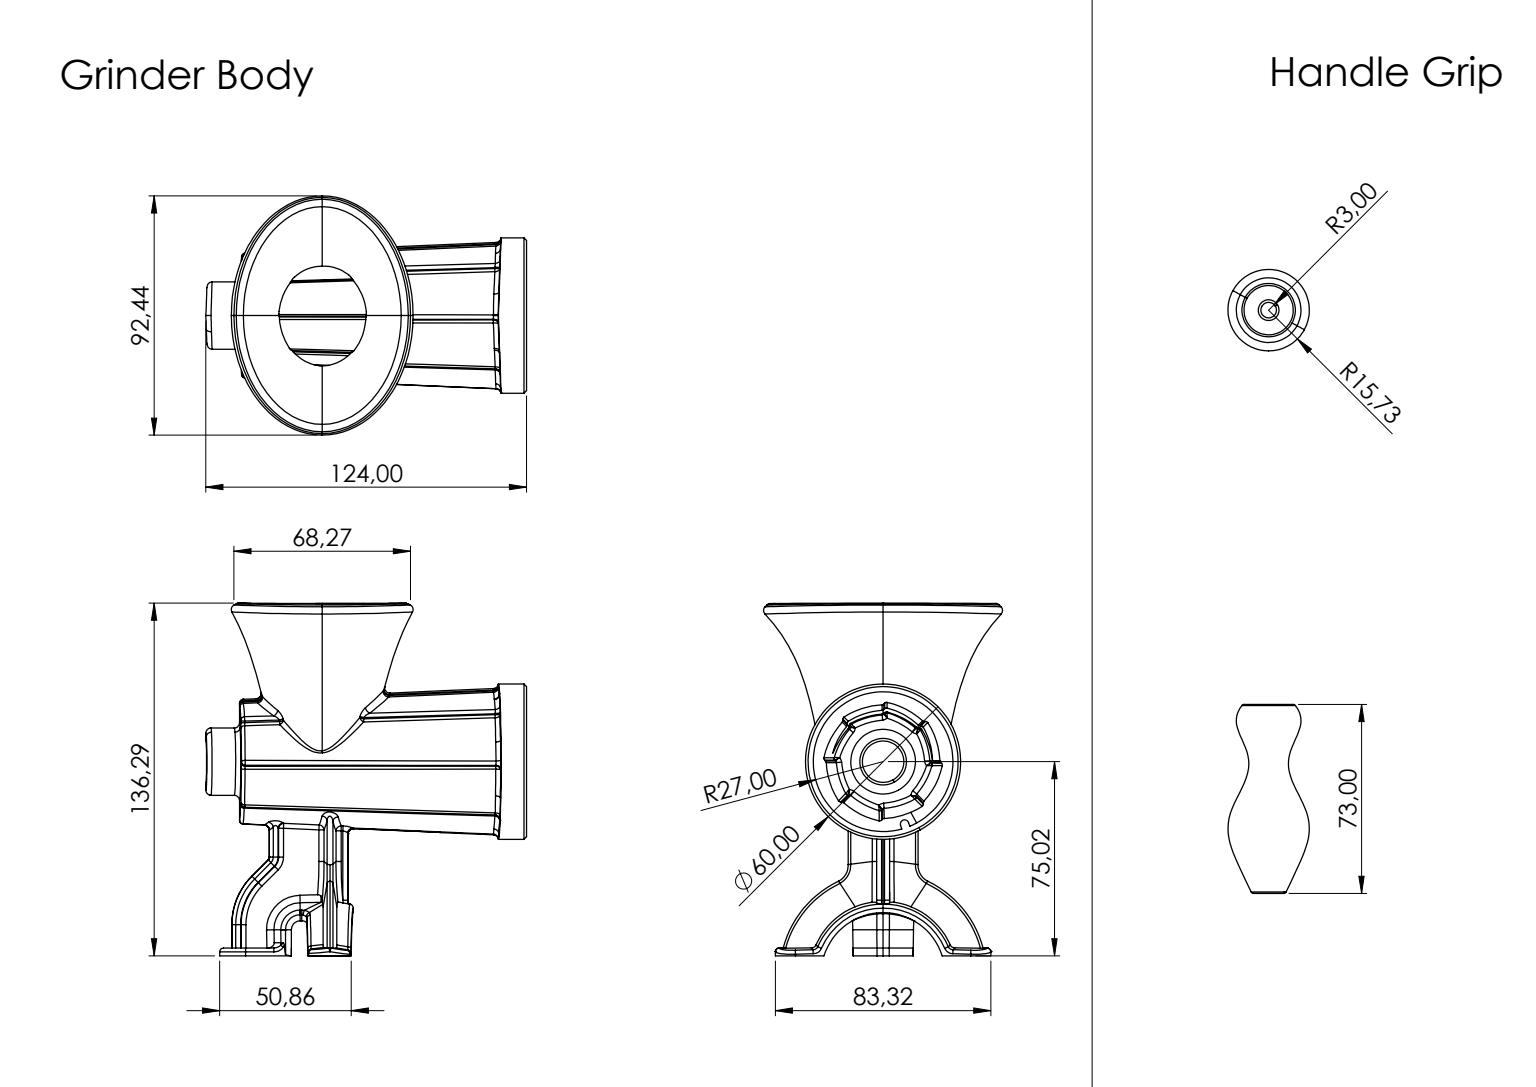
ISO-10303-21;
HEADER;
FILE_DESCRIPTION (('STEP AP214'),
    '1' );
FILE_NAME ('Handle Grip.step',
    '2026-10-06T09:49:54',
    ( '' ),
    ( '' ),
    'SwSTEP 2.0',
    'SolidWorks 2020',
    '' );
FILE_SCHEMA (( 'AUTOMOTIVE_DESIGN' ));
ENDSEC;

DATA;
#101=AXIS2_PLACEMENT_3D ( 'NONE', #52542, #86674, #33491 ) ;
#229=( LENGTH_UNIT ( ) NAMED_UNIT ( * ) SI_UNIT ( .MILLI., .METRE. ) );
#251=ORIENTED_EDGE ( 'NONE', *, *, #53107, .T. ) ;
#286=DIRECTION ( 'NONE',  ( 0.8775825618903774217, -3.365001152038843908E-31, 0.4794255386041944567 ) ) ;
#350=CARTESIAN_POINT ( 'NONE',  ( -113.4000000000000057, 1358.631207110790001, 311.1659210709989907 ) ) ;
#403=CIRCLE ( 'NONE', #27160, 5.868098490439995985 ) ;
#829=CARTESIAN_POINT ( 'NONE',  ( -113.4000000000000057, 1306.913060387289988, 304.2218459572590064 ) ) ;
#1026=AXIS2_PLACEMENT_3D ( 'NONE', #39081, #107399, #20087 ) ;
#1200=DIRECTION ( 'NONE',  ( -1.836970198721029688E-16, -1.000000000000000000, 0.000000000000000000 ) ) ;
#1407=VERTEX_POINT ( 'NONE', #25256 ) ;
#1429=CARTESIAN_POINT ( 'NONE',  ( -110.7672523143288856, 1378.813060387289852, 305.6601225730716465 ) ) ;
#1717=CARTESIAN_POINT ( 'NONE',  ( -113.4000000000000057, 1306.483669372790018, 297.4506287831990221 ) ) ;
#2006=CARTESIAN_POINT ( 'NONE',  ( -121.4211954113600029, 1309.112692017090239, 304.2218459572590064 ) ) ;
#2272=ORIENTED_EDGE ( 'NONE', *, *, #46910, .F. ) ;
#2632=VECTOR ( 'NONE', #26109, 1000.000000000000114 ) ;
#2857=VERTEX_POINT ( 'NONE', #4258 ) ;
#2858=AXIS2_PLACEMENT_3D ( 'NONE', #14026, #56057, #90747 ) ;
#2967=CARTESIAN_POINT ( 'NONE',  ( -113.4000000000000057, 1377.418846546390114, 293.0440248834589738 ) ) ;
#3089=EDGE_LOOP ( 'NONE', ( #34929, #47856, #37715, #44340, #103281 ) ) ;
#3113=CARTESIAN_POINT ( 'NONE',  ( -113.4000000000000057, 1306.483669372790018, 310.9930631313190474 ) ) ;
#3988=ORIENTED_EDGE ( 'NONE', *, *, #12337, .F. ) ;
#4058=CARTESIAN_POINT ( 'NONE',  ( -100.5161172129000136, 1371.894749952189613, 291.3379631701586732 ) ) ;
#4196=( LENGTH_UNIT ( ) NAMED_UNIT ( * ) SI_UNIT ( .MILLI., .METRE. ) );
#4258=CARTESIAN_POINT ( 'NONE',  ( -110.8380420702032580, 1377.913060387289988, 302.6609578876201567 ) ) ;
#4283=ORIENTED_EDGE ( 'NONE', *, *, #31051, .F. ) ;
#4332=CARTESIAN_POINT ( 'NONE',  ( -123.8569892972382007, 1368.558218059088176, 298.5091666679096534 ) ) ;
#4655=CARTESIAN_POINT ( 'NONE',  ( -113.4000000000000057, 1378.913060387289988, 304.2218459572590064 ) ) ;
#4738=CARTESIAN_POINT ( 'NONE',  ( -113.4000000000000057, 1377.913060387289988, 304.2218459572590064 ) ) ;
#5130=CARTESIAN_POINT ( 'NONE',  ( -113.4000000000000057, 1368.558218059089995, 292.3061701549589770 ) ) ;
#5132=DIRECTION ( 'NONE',  ( -1.836970198721029688E-16, -1.000000000000000000, 0.000000000000000000 ) ) ;
#5415=CARTESIAN_POINT ( 'NONE',  ( -124.5778210737999672, 1377.418846546389204, 315.3996670310588115 ) ) ;
#5523=ORIENTED_EDGE ( 'NONE', *, *, #44607, .T. ) ;
#5697=CARTESIAN_POINT ( 'NONE',  ( -113.4000000000000057, 1340.114449826970031, 286.9633900369479989 ) ) ;
#5970=CARTESIAN_POINT ( 'NONE',  ( -125.6580589596999431, 1375.179104070691892, 301.0918496320489339 ) ) ;
#6184=CARTESIAN_POINT ( 'NONE',  ( -113.4000000000000057, 1306.483669372790018, 304.2218459572590064 ) ) ;
#6228=CARTESIAN_POINT ( 'NONE',  ( -122.7580815721776446, 1314.643966242389979, 299.1095026942255686 ) ) ;
#6517=CARTESIAN_POINT ( 'NONE',  ( -130.6584559203111269, 1340.114449826969121, 299.8150386652596353 ) ) ;
#6581=DIRECTION ( 'NONE',  ( -0.4794255386041976763, 8.806904269216897590E-17, 0.8775825618903756453 ) ) ;
#6680=CARTESIAN_POINT ( 'NONE',  ( -102.9430107027000076, 1368.558218059089995, 309.9345252466190459 ) ) ;
#6772=CARTESIAN_POINT ( 'NONE',  ( -96.21470915085021147, 1331.448250124730293, 287.0365551081087574 ) ) ;
#6912=CARTESIAN_POINT ( 'NONE',  ( -123.3741145675100057, 1345.325269380309919, 298.7729623350389829 ) ) ;
#7070=CARTESIAN_POINT ( 'NONE',  ( -126.6653580272000283, 1320.102705746890024, 317.4872039844593132 ) ) ;
#7239=CARTESIAN_POINT ( 'NONE',  ( -107.4576978852700080, 1306.483669372790018, 307.4681403979390097 ) ) ;
#7336=CARTESIAN_POINT ( 'NONE',  ( -113.4000000000000057, 1348.229899472569969, 298.0159978832119805 ) ) ;
#7468=CARTESIAN_POINT ( 'NONE',  ( -125.0414468819000007, 1320.102705746890251, 297.8620945402790312 ) ) ;
#7518=DIRECTION ( 'NONE',  ( -1.836970198721029688E-16, -1.000000000000000000, 0.000000000000000000 ) ) ;
#7591=VERTEX_POINT ( 'NONE', #51464 ) ;
#7614=CARTESIAN_POINT ( 'NONE',  ( -119.4939992282754417, 1358.631207110788182, 300.8926790057471408 ) ) ;
#7900=ADVANCED_FACE ( 'NONE', ( #17152 ), #95557, .F. ) ;
#8015=CARTESIAN_POINT ( 'NONE',  ( -122.8636594665699988, 1366.350733876289951, 299.0518252276390285 ) ) ;
#8157=CARTESIAN_POINT ( 'NONE',  ( -125.0414468819037381, 1320.102705746890024, 297.8620945402922757 ) ) ;
#8706=DIRECTION ( 'NONE',  ( -1.836970198721029688E-16, -1.000000000000000000, -1.314768175368352060E-31 ) ) ;
#8707=CARTESIAN_POINT ( 'NONE',  ( -120.3440751137400042, 1358.631207110790001, 304.2218459572590064 ) ) ;
#8815=DIRECTION ( 'NONE',  ( -1.000000000000000000, 1.836970198721029688E-16, 0.000000000000000000 ) ) ;
#9133=APPLICATION_CONTEXT ( 'automotive_design' ) ;
#9933=PLANE ( 'NONE',  #92465 ) ;
#10275=VERTEX_POINT ( 'NONE', #42078 ) ;
#10464=EDGE_CURVE ( 'NONE', #44860, #89357, #58741, .T. ) ;
#10704=AXIS2_PLACEMENT_3D ( 'NONE', #108539, #65462, #107981 ) ;
#10869=VERTEX_POINT ( 'NONE', #110110 ) ;
#11071=DIRECTION ( 'NONE',  ( -4.648609652910299899E-17, -1.000000000000000000, 2.252106476759999926E-16 ) ) ;
#11095=AXIS2_PLACEMENT_3D ( 'NONE', #75738, #33162, #91434 ) ;
#11349=CARTESIAN_POINT ( 'NONE',  ( -101.5731991332999513, 1376.302340817389677, 292.3950450905593357 ) ) ;
#11561=CIRCLE ( 'NONE', #74167, 0.9999999999999930056 ) ;
#11756=PRODUCT_DEFINITION ( 'UNKNOWN', '', #20769, #12102 ) ;
#12085=DIRECTION ( 'NONE',  ( 0.4794255386041977873, -8.806904269216896357E-17, -0.8775825618903755343 ) ) ;
#12102=PRODUCT_DEFINITION_CONTEXT ( 'detailed design', #9133, 'design' ) ;
#12158=( GEOMETRIC_REPRESENTATION_CONTEXT ( 3 ) GLOBAL_UNCERTAINTY_ASSIGNED_CONTEXT ( ( #92795 ) ) GLOBAL_UNIT_ASSIGNED_CONTEXT ( ( #4196, #29376, #13113 ) ) REPRESENTATION_CONTEXT ( 'NONE', 'WORKASPACE' ) );
#12337=EDGE_CURVE ( 'NONE', #26502, #73768, #403, .T. ) ;
#12429=CARTESIAN_POINT ( 'NONE',  ( -101.1419410403000541, 1375.179104070690755, 291.9637869975591684 ) ) ;
#12459=ADVANCED_FACE ( 'NONE', ( #31711 ), #24972, .T. ) ;
#12466=ORIENTED_EDGE ( 'NONE', *, *, #70639, .F. ) ;
#12558=EDGE_CURVE ( 'NONE', #2857, #32152, #104036, .T. ) ;
#12715=CARTESIAN_POINT ( 'NONE',  ( -125.2268008667000743, 1376.302340817389677, 301.2019679020577883 ) ) ;
#12885=AXIS2_PLACEMENT_3D ( 'NONE', #6184, #77810, #102438 ) ;
#12969=CARTESIAN_POINT ( 'NONE',  ( -102.2221789262000016, 1377.418846546389659, 307.0760123268498205 ) ) ;
#12970=CARTESIAN_POINT ( 'NONE',  ( -113.4000000000000057, 1378.913060387289988, 304.2218459572590064 ) ) ;
#13113=( NAMED_UNIT ( * ) SI_UNIT ( $, .STERADIAN. ) SOLID_ANGLE_UNIT ( ) );
#13511=CARTESIAN_POINT ( 'NONE',  ( -102.6162175075999983, 1366.350733876289951, 304.2218459572590064 ) ) ;
#13792=CARTESIAN_POINT ( 'NONE',  ( -123.2094608542982570, 1377.418846546388068, 298.8629130685321229 ) ) ;
#14026=CARTESIAN_POINT ( 'NONE',  ( -113.4000000000000057, 1377.913060387289988, 304.2218459572590064 ) ) ;
#14069=CARTESIAN_POINT ( 'NONE',  ( -113.4000000000000057, 1358.631207110790001, 297.2777708435189652 ) ) ;
#14451=CARTESIAN_POINT ( 'NONE',  ( -115.9619579297967391, 1377.913060387289988, 305.7827340268977991 ) ) ;
#14606=MECHANICAL_DESIGN_GEOMETRIC_PRESENTATION_REPRESENTATION('',(#39642),#34280);
#14628=CARTESIAN_POINT ( 'NONE',  ( -98.25428012471454053, 1340.114449826970258, 312.4959906388990589 ) ) ;
#14643=ORIENTED_EDGE ( 'NONE', *, *, #65595, .F. ) ;
#14862=DIRECTION ( 'NONE',  ( 0.8775825618903687619, 0.000000000000000000, 0.4794255386042102218 ) ) ;
#14900=CARTESIAN_POINT ( 'NONE',  ( -113.4000000000000057, 1320.102705746890251, 317.4872039844590290 ) ) ;
#14956=DIRECTION ( 'NONE',  ( 0.8775825618903754233, 0.000000000000000000, 0.4794255386041978984 ) ) ;
#15074=ORIENTED_EDGE ( 'NONE', *, *, #108277, .F. ) ;
#15161=CARTESIAN_POINT ( 'NONE',  ( -101.4843241977000758, 1368.558218059089995, 292.3061701549589770 ) ) ;
#15290=ORIENTED_EDGE ( 'NONE', *, *, #102111, .T. ) ;
#15299=CARTESIAN_POINT ( 'NONE',  ( -127.5184075663999863, 1336.950374720429863, 296.5089247511289727 ) ) ;
#15448=CARTESIAN_POINT ( 'NONE',  ( -124.1837824923999989, 1366.350733876289951, 304.2218459572590064 ) ) ;
#15582=ORIENTED_EDGE ( 'NONE', *, *, #104815, .T. ) ;
#15601=CARTESIAN_POINT ( 'NONE',  ( -102.0933291366000049, 1371.894749952190068, 310.3987084017590519 ) ) ;
#15700=CARTESIAN_POINT ( 'NONE',  ( -104.0419184806740134, 1314.643966242388842, 309.3341893170371577 ) ) ;
#15995=CARTESIAN_POINT ( 'NONE',  ( -119.6058480740469463, 1348.229899472570878, 302.6372327872264236 ) ) ;
#16163=CARTESIAN_POINT ( 'NONE',  ( -100.0318980807000031, 1325.797319984390015, 311.5248733202390099 ) ) ;
#16227=CARTESIAN_POINT ( 'NONE',  ( -105.0428569062679145, 1377.913060387289988, 308.7873740373456144 ) ) ;
#16321=CARTESIAN_POINT ( 'NONE',  ( -113.4000000000000057, 1308.913060387289988, 304.2218459572590064 ) ) ;
#16535=CARTESIAN_POINT ( 'NONE',  ( -120.3440751137400895, 1358.631207110789774, 311.1659210709988770 ) ) ;
#16780=CARTESIAN_POINT ( 'NONE',  ( -113.4000000000000057, 1375.913060387289988, 304.2218459572590064 ) ) ;
#17081=CARTESIAN_POINT ( 'NONE',  ( -128.5457199608194401, 1340.114449826969576, 295.9477014321888646 ) ) ;
#17152=FACE_OUTER_BOUND ( 'NONE', #3089, .T. ) ;
#17255=CARTESIAN_POINT ( 'NONE',  ( -99.28159243359999664, 1336.950374720429863, 311.9347671633890400 ) ) ;
#17443=AXIS2_PLACEMENT_3D ( 'NONE', #30561, #73124, #54692 ) ;
#17475=DIRECTION ( 'NONE',  ( 9.404037925578970303E-16, -1.000000000000000000, 2.220446049250000002E-16 ) ) ;
#17505=ORIENTED_EDGE ( 'NONE', *, *, #35220, .F. ) ;
#17543=VERTEX_POINT ( 'NONE', #37700 ) ;
#17810=CARTESIAN_POINT ( 'NONE',  ( -105.2220349633299890, 1311.832804576489934, 308.6894886186490226 ) ) ;
#17819=VERTEX_POINT ( 'NONE', #74067 ) ;
#18298=DIRECTION ( 'NONE',  ( -1.836970198721029688E-16, -1.000000000000000000, 0.000000000000000000 ) ) ;
#18816=LINE ( 'NONE', #45167, #2632 ) ;
#18866=DIRECTION ( 'NONE',  ( -1.836970198721029688E-16, -1.000000000000000000, 0.000000000000000000 ) ) ;
#19178=SURFACE_STYLE_FILL_AREA ( #70212 ) ;
#19307=CARTESIAN_POINT ( 'NONE',  ( -120.1712171740600041, 1306.483669372790018, 304.2218459572590064 ) ) ;
#19407=EDGE_CURVE ( 'NONE', #20038, #77300, #65776, .T. ) ;
#19502=CARTESIAN_POINT ( 'NONE',  ( -113.4000000000000057, 1375.913060387289988, 304.2218459572590064 ) ) ;
#19593=DIRECTION ( 'NONE',  ( 0.8775825618903774217, -3.365001152038843908E-31, 0.4794255386041944567 ) ) ;
#19696=VERTEX_POINT ( 'NONE', #44493 ) ;
#20038=VERTEX_POINT ( 'NONE', #73706 ) ;
#20087=DIRECTION ( 'NONE',  ( -1.000000000000000000, 1.836970198721029688E-16, 0.000000000000000000 ) ) ;
#20173=DIRECTION ( 'NONE',  ( -1.000000000000000000, 0.000000000000000000, 0.000000000000000000 ) ) ;
#20271=CARTESIAN_POINT ( 'NONE',  ( -113.4000000000000057, 1378.528619065190014, 293.9108410952590020 ) ) ;
#20435=EDGE_CURVE ( 'NONE', #77300, #38227, #60419, .T. ) ;
#20538=ORIENTED_EDGE ( 'NONE', *, *, #12337, .T. ) ;
#20769=PRODUCT_DEFINITION_FORMATION_WITH_SPECIFIED_SOURCE ( 'ANY', '', #39314, .NOT_KNOWN. ) ;
#20819=CARTESIAN_POINT ( 'NONE',  ( -102.2221789262000726, 1377.418846546389204, 293.0440248834591443 ) ) ;
#20974=FACE_OUTER_BOUND ( 'NONE', #64827, .T. ) ;
#21092=CARTESIAN_POINT ( 'NONE',  ( -125.2268008667000174, 1376.302340817389904, 304.2218459572590064 ) ) ;
#21151=CIRCLE ( 'NONE', #57012, 0.9999999999999930056 ) ;
#21355=CARTESIAN_POINT ( 'NONE',  ( -102.6425412750940325, 1375.179104070689846, 310.0986725874599870 ) ) ;
#21632=AXIS2_PLACEMENT_3D ( 'NONE', #110085, #42890, #42328 ) ;
#21717=FACE_OUTER_BOUND ( 'NONE', #33987, .T. ) ;
#21901=CARTESIAN_POINT ( 'NONE',  ( -102.7365228771000005, 1314.643966242390206, 304.2218459572590064 ) ) ;
#22452=CARTESIAN_POINT ( 'NONE',  ( -106.4559248862599361, 1358.631207110789774, 297.2777708435190220 ) ) ;
#22482=ORIENTED_EDGE ( 'NONE', *, *, #31051, .T. ) ;
#22521=DIRECTION ( 'NONE',  ( -1.836970198721029688E-16, -1.000000000000000000, -1.314768175368352060E-31 ) ) ;
#22735=CARTESIAN_POINT ( 'NONE',  ( -103.0210057964301740, 1376.302340817391269, 309.8919163327337856 ) ) ;
#23017=CARTESIAN_POINT ( 'NONE',  ( -107.3060008061400197, 1358.631207110790911, 307.5510129717682162 ) ) ;
#23093=LINE ( 'NONE', #90859, #65252 ) ;
#23162=VECTOR ( 'NONE', #70390, 1000.000000000000227 ) ;
#23304=CARTESIAN_POINT ( 'NONE',  ( -125.3156758022999213, 1368.558218059088631, 301.1792744052535227 ) ) ;
#23576=CARTESIAN_POINT ( 'NONE',  ( -106.3607388212290061, 1309.112692017090239, 308.0674119603681902 ) ) ;
#23848=CARTESIAN_POINT ( 'NONE',  ( -107.8722023357835695, 1311.832804576487888, 313.5405874544188123 ) ) ;
#23924=LINE ( 'NONE', #48056, #38012 ) ;
#24111=CARTESIAN_POINT ( 'NONE',  ( -120.4682768577266927, 1368.558218059088176, 292.3061701549587497 ) ) ;
#24405=CARTESIAN_POINT ( 'NONE',  ( -124.1837824924000557, 1366.350733876290406, 301.4682942176205529 ) ) ;
#24627=ADVANCED_FACE ( 'NONE', ( #64326, #21717 ), #71653, .F. ) ;
#24835=AXIS2_PLACEMENT_3D ( 'NONE', #19502, #53704, #87845 ) ;
#24899=DIRECTION ( 'NONE',  ( -1.000000000000000000, 0.000000000000000000, 0.000000000000000000 ) ) ;
#24911=ORIENTED_EDGE ( 'NONE', *, *, #44245, .T. ) ;
#24939=CARTESIAN_POINT ( 'NONE',  ( -125.3156758022999924, 1368.558218059089995, 304.2218459572590064 ) ) ;
#24972=( BOUNDED_SURFACE ( )  B_SPLINE_SURFACE ( 5, 2, ( 
 ( #91066, #64807, #98915, #107324, #82679, #56385, #106226 ),
 ( #13792, #47976, #82116, #5415, #39574, #46352, #40115 ),
 ( #73747, #12715, #21092, #107871, #38462, #99457, #22735 ),
 ( #65897, #5970, #100014, #54747, #88877, #37930, #72112 ),
 ( #29510, #63703, #46899, #55295, #97813, #89425, #81023 ),
 ( #4332, #23304, #24939, #34477, #108987, #59151, #109536 ),
 ( #32810, #24405, #15448, #93804, #58039, #66995, #76477 ),
 ( #7614, #93272, #8707, #16535, #350, #83227, #85408 ),
 ( #50726, #15995, #49639, #84323, #101105, #41227, #75397 ),
 ( #17081, #6517, #25502, #67550, #50197, #40670, #42885 ),
 ( #83776, #84857, #92177, #57499, #41770, #75927, #58589 ),
 ( #8157, #32272, #42324, #7070, #14900, #66454, #74843 ),
 ( #92719, #91624, #77042, #59692, #110080, #33356, #101652 ),
 ( #51276, #110630, #100567, #33913, #68107, #23848, #102222 ),
 ( #68652, #49092, #2006, #103884, #37242, #96036, #36141 ),
 ( #104438, #35572, #19307, #35021, #3113, #79254, #26048 ) ),
 .UNSPECIFIED., .F., .F., .F. ) 
 B_SPLINE_SURFACE_WITH_KNOTS ( ( 6, 3, 3, 1, 3, 6 ),
 ( 3, 2, 2, 3 ),
 ( 0.4214913904879999951, 6.500000000000000000, 18.08975840989999995, 46.86861349480000172, 60.45619974110000072, 75.86994138869999915 ),
 ( 2.628620570832299830, 3.141592653589790007, 4.712388980384689674, 5.770213224422659160 ),
 .UNSPECIFIED. ) 
 GEOMETRIC_REPRESENTATION_ITEM ( )  RATIONAL_B_SPLINE_SURFACE ( (
 ( 0.8711730262222689980, 0.9043503973638329363, 1.000000000000000000, 0.7071067811865480168, 1.000000000000000000, 0.8027563838226099424, 0.8711730262223420507),
 ( 0.8711730262222689980, 0.9043503973638329363, 1.000000000000000000, 0.7071067811865480168, 1.000000000000000000, 0.8027563838226099424, 0.8711730262223420507),
 ( 0.8711730262222689980, 0.9043503973638329363, 1.000000000000000000, 0.7071067811865480168, 1.000000000000000000, 0.8027563838226099424, 0.8711730262223420507),
 ( 0.8711730262222689980, 0.9043503973638329363, 1.000000000000000000, 0.7071067811865480168, 1.000000000000000000, 0.8027563838226099424, 0.8711730262223420507),
 ( 0.8711730262222689980, 0.9043503973638329363, 1.000000000000000000, 0.7071067811865480168, 1.000000000000000000, 0.8027563838226099424, 0.8711730262223420507),
 ( 0.8711730262222689980, 0.9043503973638329363, 1.000000000000000000, 0.7071067811865480168, 1.000000000000000000, 0.8027563838226099424, 0.8711730262223420507),
 ( 0.8711730262222689980, 0.9043503973638329363, 1.000000000000000000, 0.7071067811865480168, 1.000000000000000000, 0.8027563838226099424, 0.8711730262223420507),
 ( 0.8711730262222689980, 0.9043503973638329363, 1.000000000000000000, 0.7071067811865480168, 1.000000000000000000, 0.8027563838226099424, 0.8711730262223420507),
 ( 0.8711730262222689980, 0.9043503973638329363, 1.000000000000000000, 0.7071067811865480168, 1.000000000000000000, 0.8027563838226099424, 0.8711730262223420507),
 ( 0.8711730262222689980, 0.9043503973638329363, 1.000000000000000000, 0.7071067811865480168, 1.000000000000000000, 0.8027563838226099424, 0.8711730262223420507),
 ( 0.8711730262222689980, 0.9043503973638329363, 1.000000000000000000, 0.7071067811865480168, 1.000000000000000000, 0.8027563838226099424, 0.8711730262223420507),
 ( 0.8711730262222689980, 0.9043503973638329363, 1.000000000000000000, 0.7071067811865480168, 1.000000000000000000, 0.8027563838226099424, 0.8711730262223420507),
 ( 0.8711730262222689980, 0.9043503973638329363, 1.000000000000000000, 0.7071067811865480168, 1.000000000000000000, 0.8027563838226099424, 0.8711730262223420507),
 ( 0.8711730262222689980, 0.9043503973638329363, 1.000000000000000000, 0.7071067811865480168, 1.000000000000000000, 0.8027563838226099424, 0.8711730262223420507),
 ( 0.8711730262222689980, 0.9043503973638329363, 1.000000000000000000, 0.7071067811865480168, 1.000000000000000000, 0.8027563838226099424, 0.8711730262223420507),
 ( 0.8711730262222689980, 0.9043503973638329363, 1.000000000000000000, 0.7071067811865480168, 1.000000000000000000, 0.8027563838226099424, 0.8711730262223420507) ) ) 
 REPRESENTATION_ITEM ( '' )  SURFACE ( )  );
#25213=CARTESIAN_POINT ( 'NONE',  ( -113.4000000000000057, 1309.112692017090239, 296.2006505458990091 ) ) ;
#25256=CARTESIAN_POINT ( 'NONE',  ( -119.3423021147300034, 1306.483669372790018, 300.9755515165790030 ) ) ;
#25349=CARTESIAN_POINT ( 'NONE',  ( -127.3242238164999947, 1328.501055712589960, 296.6150078171390305 ) ) ;
#25444=EDGE_CURVE ( 'NONE', #10869, #2857, #51125, .T. ) ;
#25502=CARTESIAN_POINT ( 'NONE',  ( -130.6584559203110132, 1340.114449826970031, 304.2218459572590064 ) ) ;
#25523=ORIENTED_EDGE ( 'NONE', *, *, #12558, .T. ) ;
#26048=CARTESIAN_POINT ( 'NONE',  ( -107.4576978852700648, 1306.483669372788427, 307.4681403979344623 ) ) ;
#26109=DIRECTION ( 'NONE',  ( -0.6038592750913972518, 0.7071067811868648745, 0.3679048462383220919 ) ) ;
#26295=DIRECTION ( 'NONE',  ( 0.4794255386042002298, -8.806904269216945661E-17, -0.8775825618903744241 ) ) ;
#26502=VERTEX_POINT ( 'NONE', #109208 ) ;
#26555=DIRECTION ( 'NONE',  ( -4.222254822704919979E-17, -1.000000000000000000, 7.728785610902649958E-17 ) ) ;
#27122=CONICAL_SURFACE ( 'NONE', #39661, 0.9999999999999956701, 0.7853981633970000820 ) ;
#27160=AXIS2_PLACEMENT_3D ( 'NONE', #68239, #59824, #77175 ) ;
#27610=SHAPE_REPRESENTATION_RELATIONSHIP ( 'NONE' , 'NONE' ,  #45156, #67999 ) ;
#27847=CARTESIAN_POINT ( 'NONE',  ( -106.8999999999999915, 1305.913060387289988, 304.2218459572590064 ) ) ;
#28228=STYLED_ITEM ( 'NONE', ( #87654 ), #46097 ) ;
#28303=EDGE_CURVE ( 'NONE', #17819, #38227, #106482, .T. ) ;
#28529=AXIS2_PLACEMENT_3D ( 'NONE', #4738, #98798, #105568 ) ;
#28846=FILL_AREA_STYLE_COLOUR ( '', #76500 ) ;
#28896=CIRCLE ( 'NONE', #44985, 0.9999999999999930056 ) ;
#28917=UNCERTAINTY_MEASURE_WITH_UNIT (LENGTH_MEASURE( 1.000000000000000082E-05 ), #80223, 'distance_accuracy_value', 'NONE');
#28977=DIRECTION ( 'NONE',  ( -1.000000000000000000, 0.000000000000000000, 0.000000000000000000 ) ) ;
#29376=( NAMED_UNIT ( * ) PLANE_ANGLE_UNIT ( ) SI_UNIT ( $, .RADIAN. ) );
#29510=CARTESIAN_POINT ( 'NONE',  ( -124.7066708633992391, 1371.894749952189386, 298.0449835127411689 ) ) ;
#29511=EDGE_CURVE ( 'NONE', #38227, #17543, #42104, .T. ) ;
#29747=ORIENTED_EDGE ( 'NONE', *, *, #82319, .T. ) ;
#29782=CARTESIAN_POINT ( 'NONE',  ( -103.0889951380000156, 1378.528619065190696, 293.9108410952588883 ) ) ;
#30156=ORIENTED_EDGE ( 'NONE', *, *, #108277, .T. ) ;
#30561=CARTESIAN_POINT ( 'NONE',  ( -113.4000000000000057, 1378.913060387289988, 304.2218459572590064 ) ) ;
#30575=CYLINDRICAL_SURFACE ( 'NONE', #90237, 3.000000000000017764 ) ;
#30696=ORIENTED_EDGE ( 'NONE', *, *, #65845, .T. ) ;
#30877=CARTESIAN_POINT ( 'NONE',  ( -122.8636594665523489, 1366.350733876290178, 299.0518252276563658 ) ) ;
#30977=EDGE_CURVE ( 'NONE', #81044, #19696, #18816, .T. ) ;
#31051=EDGE_CURVE ( 'NONE', #17819, #73768, #11561, .T. ) ;
#31052=ORIENTED_EDGE ( 'NONE', *, *, #65845, .F. ) ;
#31430=CARTESIAN_POINT ( 'NONE',  ( -107.1941519259529230, 1348.229899472571105, 305.8064591614598839 ) ) ;
#31711=FACE_OUTER_BOUND ( 'NONE', #80783, .T. ) ;
#31985=CARTESIAN_POINT ( 'NONE',  ( -113.4000000000000057, 1311.832804576489934, 294.9031044600990299 ) ) ;
#32123=CARTESIAN_POINT ( 'NONE',  ( -119.0092909768300018, 1350.849221539110204, 301.1574763303589748 ) ) ;
#32152=VERTEX_POINT ( 'NONE', #63754 ) ;
#32272=CARTESIAN_POINT ( 'NONE',  ( -126.6653580271998862, 1320.102705746891161, 300.8346439529095164 ) ) ;
#32545=CARTESIAN_POINT ( 'NONE',  ( -98.31848851494262931, 1331.448250124730066, 312.4609134345859047 ) ) ;
#32810=CARTESIAN_POINT ( 'NONE',  ( -122.8636594665494499, 1366.350733876287677, 299.0518252276506814 ) ) ;
#32974=CARTESIAN_POINT ( 'NONE',  ( -107.3060007717200079, 1358.631207110790001, 307.5510129087689961 ) ) ;
#33078=CARTESIAN_POINT ( 'NONE',  ( -103.9363405868959518, 1366.350733876290633, 309.3918667846981521 ) ) ;
#33145=EDGE_CURVE ( 'NONE', #2857, #7591, #23924, .T. ) ;
#33162=DIRECTION ( 'NONE',  ( -1.836970198721029688E-16, -1.000000000000000000, 0.000000000000000000 ) ) ;
#33215=CARTESIAN_POINT ( 'NONE',  ( -122.4487580624700058, 1378.528619065190014, 299.2784868977390147 ) ) ;
#33356=CARTESIAN_POINT ( 'NONE',  ( -107.0745166769187335, 1314.643966242389979, 314.8853230801587415 ) ) ;
#33491=DIRECTION ( 'NONE',  ( -1.000000000000000000, 0.000000000000000000, 0.000000000000000000 ) ) ;
#33513=CARTESIAN_POINT ( 'NONE',  ( -104.3512419375300055, 1378.528619065190014, 309.1652050167789980 ) ) ;
#33657=AXIS2_PLACEMENT_3D ( 'NONE', #94224, #69069, #42188 ) ;
#33913=CARTESIAN_POINT ( 'NONE',  ( -122.7187414971600390, 1311.832804576490389, 313.5405874544188691 ) ) ;
#33987=EDGE_LOOP ( 'NONE', ( #15074, #51270 ) ) ;
#34206=CLOSED_SHELL ( 'NONE', ( #74966, #61184, #92370, #7900, #41766, #53548, #66841, #98059, #103639, #24627, #76834, #93325, #12459, #91525 ) ) ;
#34280=( GEOMETRIC_REPRESENTATION_CONTEXT ( 3 ) GLOBAL_UNCERTAINTY_ASSIGNED_CONTEXT ( ( #28917 ) ) GLOBAL_UNIT_ASSIGNED_CONTEXT ( ( #80223, #71870, #80776 ) ) REPRESENTATION_CONTEXT ( 'NONE', 'WORKASPACE' ) );
#34339=ORIENTED_EDGE ( 'NONE', *, *, #33145, .T. ) ;
#34477=CARTESIAN_POINT ( 'NONE',  ( -125.3156758023000918, 1368.558218059089995, 316.1375217595589220 ) ) ;
#34541=CARTESIAN_POINT ( 'NONE',  ( -113.4000000000000057, 1378.813060387289852, 304.2218459572590064 ) ) ;
#34564=CARTESIAN_POINT ( 'NONE',  ( -113.4000000000000057, 1305.913060387289988, 304.2218459572590064 ) ) ;
#34643=CARTESIAN_POINT ( 'NONE',  ( -103.4258854324899914, 1345.325269380309919, 309.6707295794789729 ) ) ;
#34739=CARTESIAN_POINT ( 'NONE',  ( -107.4576979188310162, 1306.483669372790018, 307.4681404593670777 ) ) ;
#34929=ORIENTED_EDGE ( 'NONE', *, *, #25444, .F. ) ;
#35021=CARTESIAN_POINT ( 'NONE',  ( -120.1712171740600326, 1306.483669372790246, 310.9930631313191043 ) ) ;
#35220=EDGE_CURVE ( 'NONE', #17819, #1407, #48666, .T. ) ;
#35323=ORIENTED_EDGE ( 'NONE', *, *, #105278, .F. ) ;
#35572=CARTESIAN_POINT ( 'NONE',  ( -120.1712171740599473, 1306.483669372790928, 302.4928703550302203 ) ) ;
#35647=UNCERTAINTY_MEASURE_WITH_UNIT (LENGTH_MEASURE( 1.000000000000000082E-05 ), #229, 'distance_accuracy_value', 'NONE');
#35686=FACE_BOUND ( 'NONE', #108423, .T. ) ;
#35856=CARTESIAN_POINT ( 'NONE',  ( -118.1581044363824731, 1309.112692017089103, 296.2006505458993502 ) ) ;
#35876=DIRECTION ( 'NONE',  ( -0.4794255386042000078, 8.806904269216944428E-17, 0.8775825618903743131 ) ) ;
#36141=CARTESIAN_POINT ( 'NONE',  ( -106.3607387814725911, 1309.112692017088648, 308.0674118875946874 ) ) ;
#36160=ORIENTED_EDGE ( 'NONE', *, *, #35220, .T. ) ;
#36206=LINE ( 'NONE', #43510, #23162 ) ;
#36560=( NAMED_UNIT ( * ) PLANE_ANGLE_UNIT ( ) SI_UNIT ( $, .RADIAN. ) );
#37111=( NAMED_UNIT ( * ) SI_UNIT ( $, .STERADIAN. ) SOLID_ANGLE_UNIT ( ) );
#37207=FACE_OUTER_BOUND ( 'NONE', #75821, .T. ) ;
#37242=CARTESIAN_POINT ( 'NONE',  ( -113.4000000000000057, 1309.112692017090239, 312.2430413686190036 ) ) ;
#37700=CARTESIAN_POINT ( 'NONE',  ( -122.4487580624700058, 1378.528619065190014, 299.2784868977390147 ) ) ;
#37715=ORIENTED_EDGE ( 'NONE', *, *, #93623, .T. ) ;
#37924=EDGE_LOOP ( 'NONE', ( #108288, #20538 ) ) ;
#37930=CARTESIAN_POINT ( 'NONE',  ( -106.1286243849658177, 1375.179104070688027, 316.4799049169590717 ) ) ;
#38012=VECTOR ( 'NONE', #73821, 999.9999999999998863 ) ;
#38195=ORIENTED_EDGE ( 'NONE', *, *, #29511, .T. ) ;
#38227=VERTEX_POINT ( 'NONE', #76475 ) ;
#38462=CARTESIAN_POINT ( 'NONE',  ( -113.4000000000000057, 1376.302340817389904, 316.0486468239590181 ) ) ;
#38658=ORIENTED_EDGE ( 'NONE', *, *, #20435, .F. ) ;
#39071=AXIS2_PLACEMENT_3D ( 'NONE', #4655, #75180, #91421 ) ;
#39081=CARTESIAN_POINT ( 'NONE',  ( -103.4000000000000057, 1378.913060387289988, 304.2218459572590064 ) ) ;
#39286=CARTESIAN_POINT ( 'NONE',  ( -118.8461440515266929, 1348.229899472570651, 301.2466039018671609 ) ) ;
#39314=PRODUCT ( 'Handle Grip', 'Handle Grip', '', ( #73484 ) ) ;
#39478=EDGE_LOOP ( 'NONE', ( #95080, #25523, #60146, #42896, #31052 ) ) ;
#39568=ORIENTED_EDGE ( 'NONE', *, *, #93623, .F. ) ;
#39574=CARTESIAN_POINT ( 'NONE',  ( -113.4000000000000057, 1377.418846546390114, 315.3996670310589820 ) ) ;
#39576=EDGE_CURVE ( 'NONE', #10869, #41956, #23093, .T. ) ;
#39642=STYLED_ITEM ( 'NONE', ( #55041 ), #67999 ) ;
#39661=AXIS2_PLACEMENT_3D ( 'NONE', #16780, #69459, #49882 ) ;
#39842=CARTESIAN_POINT ( 'NONE',  ( -102.7365228771000574, 1314.643966242390661, 306.9446787514269204 ) ) ;
#40115=CARTESIAN_POINT ( 'NONE',  ( -103.5905391456986706, 1377.418846546389432, 309.5807788459800349 ) ) ;
#40274=CARTESIAN_POINT ( 'NONE',  ( -105.0428569062679145, 1378.913060387289988, 308.7873740373456144 ) ) ;
#40383=CARTESIAN_POINT ( 'NONE',  ( -125.0414468819076461, 1320.102705746891161, 297.8620945402992106 ) ) ;
#40670=CARTESIAN_POINT ( 'NONE',  ( -103.1624317239240867, 1340.114449826968666, 321.4803018775698433 ) ) ;
#40732=AXIS2_PLACEMENT_3D ( 'NONE', #16227, #26295, #42014 ) ;
#40834=CARTESIAN_POINT ( 'NONE',  ( -107.7907090231699954, 1350.849221539110204, 307.2862155841589811 ) ) ;
#40841=ORIENTED_EDGE ( 'NONE', *, *, #105278, .T. ) ;
#40936=CARTESIAN_POINT ( 'NONE',  ( -100.1346419727999972, 1320.102705746890251, 304.2218459572590064 ) ) ;
#41003=AXIS2_PLACEMENT_3D ( 'NONE', #87490, #17475, #103148 ) ;
#41069=CARTESIAN_POINT ( 'NONE',  ( -119.4939992282800034, 1358.631207110790001, 300.8926790057490166 ) ) ;
#41101=B_SPLINE_CURVE_WITH_KNOTS ( 'NONE', 5,
 ( #100960, #65738, #92564, #76894, #7468, #102066, #25349, #15299, #6912, #32123, #41069, #8015, #84168, #75784, #57355, #67404, #91480, #33215 ),
 .UNSPECIFIED., .F., .F.,
 ( 6, 3, 3, 3, 3, 6 ),
 ( -75.86994138869999915, -60.45619974110000072, -46.86861349480000172, -18.08975840989999284, -6.500000000000000000, -0.4214913904880006612 ),
 .UNSPECIFIED. ) ;
#41227=CARTESIAN_POINT ( 'NONE',  ( -109.7187440601658466, 1348.229899472568604, 310.4276940313056343 ) ) ;
#41399=CARTESIAN_POINT ( 'NONE',  ( -99.47577618349998829, 1328.501055712589960, 311.8286840973790390 ) ) ;
#41500=CARTESIAN_POINT ( 'NONE',  ( -96.14154407968899818, 1340.114449826970940, 286.9633900369476578 ) ) ;
#41766=ADVANCED_FACE ( 'NONE', ( #62881 ), #89285, .F. ) ;
#41770=CARTESIAN_POINT ( 'NONE',  ( -113.4000000000000057, 1331.448250124730066, 321.4071368064089711 ) ) ;
#41956=VERTEX_POINT ( 'NONE', #52513 ) ;
#42014=DIRECTION ( 'NONE',  ( -0.8775825618903754233, 0.000000000000000000, -0.4794255386041978984 ) ) ;
#42078=CARTESIAN_POINT ( 'NONE',  ( -116.9103302475592301, 1305.913060387289988, 302.3041438028434413 ) ) ;
#42104=CIRCLE ( 'NONE', #54674, 10.31100486199999722 ) ;
#42188=DIRECTION ( 'NONE',  ( -1.000000000000000000, 0.000000000000000000, 0.000000000000000000 ) ) ;
#42318=ORIENTED_EDGE ( 'NONE', *, *, #46910, .T. ) ;
#42324=CARTESIAN_POINT ( 'NONE',  ( -126.6653580271999999, 1320.102705746890251, 304.2218459572590064 ) ) ;
#42328=DIRECTION ( 'NONE',  ( 1.000000000000000000, 0.000000000000000000, 0.000000000000000000 ) ) ;
#42631=CIRCLE ( 'NONE', #33657, 10.31100486199999722 ) ;
#42838=TOROIDAL_SURFACE ( 'NONE', #28529, 9.522913805089999073, 1.000000000000000000 ) ;
#42885=CARTESIAN_POINT ( 'NONE',  ( -98.25428003917552644, 1340.114449826969576, 312.4959904823201100 ) ) ;
#42890=DIRECTION ( 'NONE',  ( 0.000000000000000000, 0.000000000000000000, 1.000000000000000000 ) ) ;
#42896=ORIENTED_EDGE ( 'NONE', *, *, #30977, .T. ) ;
#42979=DIRECTION ( 'NONE',  ( -1.000000000000000000, 0.000000000000000000, 0.000000000000000000 ) ) ;
#43510=CARTESIAN_POINT ( 'NONE',  ( -114.2775825618903696, 1308.913060387289988, 303.7424204186547740 ) ) ;
#44245=EDGE_CURVE ( 'NONE', #81044, #10869, #58749, .T. ) ;
#44340=ORIENTED_EDGE ( 'NONE', *, *, #44607, .F. ) ;
#44493=CARTESIAN_POINT ( 'NONE',  ( -116.8159439063953045, 1378.913060387289988, 306.3030300501105785 ) ) ;
#44607=EDGE_CURVE ( 'NONE', #32152, #44860, #69766, .T. ) ;
#44860=VERTEX_POINT ( 'NONE', #59560 ) ;
#44964=CARTESIAN_POINT ( 'NONE',  ( -113.4000000000000057, 1375.179104070690073, 291.9637869975589979 ) ) ;
#44968=AXIS2_PLACEMENT_3D ( 'NONE', #88718, #97112, #89800 ) ;
#44985=AXIS2_PLACEMENT_3D ( 'NONE', #90574, #6581, #14956 ) ;
#45156=SHAPE_REPRESENTATION ( 'Handle Grip', ( #21632 ), #71657 ) ;
#45167=CARTESIAN_POINT ( 'NONE',  ( -114.2539859765994237, 1375.913060387289988, 304.7421419804722404 ) ) ;
#45395=CARTESIAN_POINT ( 'NONE',  ( -121.7571430937320827, 1377.913060387289988, 299.6563178771723415 ) ) ;
#46064=CARTESIAN_POINT ( 'NONE',  ( -123.7789942035696811, 1376.302340817388313, 298.5517755817839998 ) ) ;
#46097=MANIFOLD_SOLID_BREP ( 'Stock-MAS-682-1', #34206 ) ;
#46352=CARTESIAN_POINT ( 'NONE',  ( -106.7694122493245175, 1377.418846546389432, 315.3996670310588115 ) ) ;
#46724=TOROIDAL_SURFACE ( 'NONE', #44968, 9.522913805089999073, 1.000000000000000000 ) ;
#46881=CIRCLE ( 'NONE', #89773, 3.000000000000002665 ) ;
#46899=CARTESIAN_POINT ( 'NONE',  ( -126.2838827870999836, 1371.894749952190068, 304.2218459572590064 ) ) ;
#46910=EDGE_CURVE ( 'NONE', #44860, #41956, #67646, .T. ) ;
#47153=DIRECTION ( 'NONE',  ( -1.000000000000000000, 0.000000000000000000, 0.000000000000000000 ) ) ;
#47699=CARTESIAN_POINT ( 'NONE',  ( -102.6162175075999414, 1366.350733876289723, 293.4380634648590558 ) ) ;
#47856=ORIENTED_EDGE ( 'NONE', *, *, #39576, .T. ) ;
#47971=EDGE_CURVE ( 'NONE', #19696, #7591, #56933, .T. ) ;
#47976=CARTESIAN_POINT ( 'NONE',  ( -124.5778210738000809, 1377.418846546389886, 301.3676796492106860 ) ) ;
#47987=ORIENTED_EDGE ( 'NONE', *, *, #55500, .T. ) ;
#48056=CARTESIAN_POINT ( 'NONE',  ( -112.5460140234005735, 1375.913060387289988, 303.7015499340457723 ) ) ;
#48258=CARTESIAN_POINT ( 'NONE',  ( -100.1346419727999688, 1320.102705746890024, 290.9564879300593248 ) ) ;
#48666=CIRCLE ( 'NONE', #11095, 6.771217174059998456 ) ;
#48815=CARTESIAN_POINT ( 'NONE',  ( -119.7968474381516302, 1366.350733876288814, 293.4380634648589989 ) ) ;
#48841=SHAPE_DEFINITION_REPRESENTATION ( #87531, #45156 ) ;
#49092=CARTESIAN_POINT ( 'NONE',  ( -121.4211954113599461, 1309.112692017089330, 302.1736985104333257 ) ) ;
#49352=CARTESIAN_POINT ( 'NONE',  ( -104.0812585028399866, 1311.832804576489934, 306.6013113658122506 ) ) ;
#49639=CARTESIAN_POINT ( 'NONE',  ( -119.6058480740470031, 1348.229899472569969, 304.2218459572590064 ) ) ;
#49798=DIRECTION ( 'NONE',  ( 0.6205445805634681733, -0.7071067811868637643, 0.3390050494208930454 ) ) ;
#49806=CARTESIAN_POINT ( 'NONE',  ( -106.3607387814799949, 1309.112692017090239, 308.0674118875990075 ) ) ;
#49882=DIRECTION ( 'NONE',  ( -0.8539859765994315399, 0.000000000000000000, 0.5202960232132425311 ) ) ;
#49903=CARTESIAN_POINT ( 'NONE',  ( -117.0812559398341222, 1348.229899472569286, 298.0159978832119236 ) ) ;
#50073=ORIENTED_EDGE ( 'NONE', *, *, #82319, .F. ) ;
#50197=CARTESIAN_POINT ( 'NONE',  ( -113.4000000000000057, 1340.114449826970031, 321.4803018775700139 ) ) ;
#50726=CARTESIAN_POINT ( 'NONE',  ( -118.8461440515248171, 1348.229899472569514, 301.2466039018639208 ) ) ;
#50902=CARTESIAN_POINT ( 'NONE',  ( -103.5905391456900020, 1377.418846546390114, 309.5807788459990206 ) ) ;
#51003=CARTESIAN_POINT ( 'NONE',  ( -120.4392612185272213, 1309.112692017090239, 300.3762800269232116 ) ) ;
#51125=CIRCLE ( 'NONE', #2858, 3.000000000000002665 ) ;
#51270=ORIENTED_EDGE ( 'NONE', *, *, #19407, .F. ) ;
#51276=CARTESIAN_POINT ( 'NONE',  ( -121.5779650366722535, 1311.832804576488343, 299.7542032958708091 ) ) ;
#51464=CARTESIAN_POINT ( 'NONE',  ( -109.9840560936046927, 1378.913060387289988, 302.1406618644074342 ) ) ;
#51534=ORIENTED_EDGE ( 'NONE', *, *, #19407, .T. ) ;
#51549=CARTESIAN_POINT ( 'NONE',  ( -117.4166280489782253, 1306.483669372789336, 297.4506287831988516 ) ) ;
#52010=CARTESIAN_POINT ( 'NONE',  ( -101.7585531180999965, 1320.102705746890251, 310.5815973742389815 ) ) ;
#52244=CIRCLE ( 'NONE', #12885, 6.771217174059998456 ) ;
#52513=CARTESIAN_POINT ( 'NONE',  ( -116.0327476856695341, 1306.913060387289988, 302.7835693414472189 ) ) ;
#52542=CARTESIAN_POINT ( 'NONE',  ( -113.4000000000000057, 1378.913060387289988, 304.2218459572590064 ) ) ;
#52726=DIRECTION ( 'NONE',  ( 0.8775825618903754233, 0.000000000000000000, 0.4794255386041978984 ) ) ;
#53107=EDGE_CURVE ( 'NONE', #1407, #26502, #28896, .T. ) ;
#53359=CARTESIAN_POINT ( 'NONE',  ( -124.7066708634027208, 1371.894749952188477, 298.0449835127481037 ) ) ;
#53548=ADVANCED_FACE ( 'NONE', ( #94148 ), #107527, .F. ) ;
#53704=DIRECTION ( 'NONE',  ( 4.057416247971030182E-16, 1.000000000000000000, -4.440892098500000003E-16 ) ) ;
#53929=FACE_OUTER_BOUND ( 'NONE', #81096, .T. ) ;
#53953=SURFACE_SIDE_STYLE ('',( #19178 ) ) ;
#54472=CARTESIAN_POINT ( 'NONE',  ( -120.0305877506754513, 1377.418846546390341, 293.0440248834586896 ) ) ;
#54674=AXIS2_PLACEMENT_3D ( 'NONE', #62787, #1200, #20173 ) ;
#54692=DIRECTION ( 'NONE',  ( -1.000000000000000000, 0.000000000000000000, 0.000000000000000000 ) ) ;
#54747=CARTESIAN_POINT ( 'NONE',  ( -125.6580589596999431, 1375.179104070690755, 316.4799049169587306 ) ) ;
#54847=ORIENTED_EDGE ( 'NONE', *, *, #28303, .T. ) ;
#55016=CARTESIAN_POINT ( 'NONE',  ( -101.5731991332999513, 1376.302340817389677, 307.2417240775760092 ) ) ;
#55041=PRESENTATION_STYLE_ASSIGNMENT (( #97033 ) ) ;
#55295=CARTESIAN_POINT ( 'NONE',  ( -126.2838827870999836, 1371.894749952189613, 317.1057287443592827 ) ) ;
#55500=EDGE_CURVE ( 'NONE', #1407, #17819, #52244, .T. ) ;
#55562=CARTESIAN_POINT ( 'NONE',  ( -102.0933292004540220, 1371.894749952189613, 310.3987085186598165 ) ) ;
#55779=CARTESIAN_POINT ( 'NONE',  ( -108.2502590933346198, 1306.913060387289988, 307.0351622366206357 ) ) ;
#56057=DIRECTION ( 'NONE',  ( -4.648609652910299899E-17, -1.000000000000000000, 2.252106476759999926E-16 ) ) ;
#56098=CARTESIAN_POINT ( 'NONE',  ( -104.0812585028399582, 1311.832804576490389, 294.9031044600990867 ) ) ;
#56355=EDGE_LOOP ( 'NONE', ( #104692, #2272, #89177, #107319 ) ) ;
#56385=CARTESIAN_POINT ( 'NONE',  ( -107.2836002040342152, 1378.528619065189787, 314.5328508192586128 ) ) ;
#56466=ORIENTED_EDGE ( 'NONE', *, *, #39576, .F. ) ;
#56653=CARTESIAN_POINT ( 'NONE',  ( -123.6375682760757115, 1340.114449826969576, 286.9633900369482831 ) ) ;
#56852=CARTESIAN_POINT ( 'NONE',  ( -109.8896697524407671, 1305.913060387289988, 306.1395481116745145 ) ) ;
#56933=CIRCLE ( 'NONE', #39071, 4.000000000000003553 ) ;
#57012=AXIS2_PLACEMENT_3D ( 'NONE', #45395, #35876, #96882 ) ;
#57171=AXIS2_PLACEMENT_3D ( 'NONE', #106584, #64058, #98177 ) ;
#57221=CARTESIAN_POINT ( 'NONE',  ( -117.5191658986970253, 1358.631207110789092, 297.2777708435188515 ) ) ;
#57355=CARTESIAN_POINT ( 'NONE',  ( -124.1574587857000012, 1375.179104070690073, 298.3450194382389782 ) ) ;
#57499=CARTESIAN_POINT ( 'NONE',  ( -130.5852908491499136, 1331.448250124730293, 321.4071368064091985 ) ) ;
#57769=CARTESIAN_POINT ( 'NONE',  ( -105.3788045886400369, 1309.112692017090239, 306.2699934482469075 ) ) ;
#58039=CARTESIAN_POINT ( 'NONE',  ( -113.4000000000000057, 1366.350733876289951, 315.0056284496589569 ) ) ;
#58303=CARTESIAN_POINT ( 'NONE',  ( -107.1941519259530082, 1348.229899472569969, 304.2218459572590064 ) ) ;
#58550=CARTESIAN_POINT ( 'NONE',  ( -113.4000000000000057, 1305.913060387289988, 304.2218459572590064 ) ) ;
#58589=CARTESIAN_POINT ( 'NONE',  ( -98.31848842976613412, 1331.448250124729157, 312.4609132786720807 ) ) ;
#58741=LINE ( 'NONE', #73897, #66884 ) ;
#58749=CIRCLE ( 'NONE', #64132, 3.000000000000002665 ) ;
#58882=ORIENTED_EDGE ( 'NONE', *, *, #28303, .F. ) ;
#59151=CARTESIAN_POINT ( 'NONE',  ( -106.3317231422732476, 1368.558218059090223, 316.1375217595586946 ) ) ;
#59560=CARTESIAN_POINT ( 'NONE',  ( -110.7672523143304488, 1306.913060387289988, 305.6601225730707370 ) ) ;
#59692=CARTESIAN_POINT ( 'NONE',  ( -124.0634771229000393, 1314.643966242389752, 314.8853230801590257 ) ) ;
#59817=AXIS2_PLACEMENT_3D ( 'NONE', #12970, #5132, #47153 ) ;
#59824=DIRECTION ( 'NONE',  ( -1.836970198721029688E-16, -1.000000000000000000, 0.000000000000000000 ) ) ;
#60146=ORIENTED_EDGE ( 'NONE', *, *, #70639, .T. ) ;
#60419=CIRCLE ( 'NONE', #40732, 0.9999999999999930056 ) ;
#60518=CARTESIAN_POINT ( 'NONE',  ( -105.3788045886400511, 1309.112692017089785, 296.2006505458987249 ) ) ;
#61184=ADVANCED_FACE ( 'NONE', ( #95430 ), #102685, .T. ) ;
#61484=EDGE_LOOP ( 'NONE', ( #72628, #30696 ) ) ;
#62100=ORIENTED_EDGE ( 'NONE', *, *, #44245, .F. ) ;
#62101=FACE_OUTER_BOUND ( 'NONE', #39478, .T. ) ;
#62188=CARTESIAN_POINT ( 'NONE',  ( -113.4000000000000057, 1306.913060387289988, 304.2218459572590064 ) ) ;
#62787=CARTESIAN_POINT ( 'NONE',  ( -113.4000000000000057, 1378.528619065190014, 304.2218459572590064 ) ) ;
#62803=AXIS2_PLACEMENT_3D ( 'NONE', #34564, #18298, #42979 ) ;
#62881=FACE_OUTER_BOUND ( 'NONE', #87056, .T. ) ;
#63041=SURFACE_STYLE_FILL_AREA ( #106098 ) ;
#63429=CARTESIAN_POINT ( 'NONE',  ( -103.5905392011000856, 1377.418846546391933, 309.5807789473911384 ) ) ;
#63703=CARTESIAN_POINT ( 'NONE',  ( -126.2838827870999836, 1371.894749952190750, 300.9320505736152427 ) ) ;
#63754=CARTESIAN_POINT ( 'NONE',  ( -110.7672523143288998, 1377.913060387289988, 305.6601225730716465 ) ) ;
#63969=CARTESIAN_POINT ( 'NONE',  ( -103.0889951380000014, 1378.528619065190014, 304.2218459572590064 ) ) ;
#64058=DIRECTION ( 'NONE',  ( -1.836970198721029688E-16, -1.000000000000000000, 0.000000000000000000 ) ) ;
#64132=AXIS2_PLACEMENT_3D ( 'NONE', #87789, #11071, #28977 ) ;
#64326=FACE_BOUND ( 'NONE', #61484, .T. ) ;
#64518=CARTESIAN_POINT ( 'NONE',  ( -100.5161172128999993, 1371.894749952190068, 304.2218459572590064 ) ) ;
#64807=CARTESIAN_POINT ( 'NONE',  ( -123.7110048620000242, 1378.528619065189332, 301.5890141660771064 ) ) ;
#64827=EDGE_LOOP ( 'NONE', ( #30156, #15290, #109079, #38658 ) ) ;
#65057=CARTESIAN_POINT ( 'NONE',  ( -106.4559248862600072, 1358.631207110790001, 304.2218459572590064 ) ) ;
#65252=VECTOR ( 'NONE', #22521, 1000.000000000000000 ) ;
#65303=CARTESIAN_POINT ( 'NONE',  ( -113.4000000000000057, 1378.813060387289852, 304.2218459572590064 ) ) ;
#65462=DIRECTION ( 'NONE',  ( -4.648609652910299899E-17, -1.000000000000000000, 2.252106476759999926E-16 ) ) ;
#65595=EDGE_CURVE ( 'NONE', #1407, #17543, #41101, .T. ) ;
#65612=CARTESIAN_POINT ( 'NONE',  ( -101.4843241977000474, 1368.558218059090905, 307.2644175748700377 ) ) ;
#65738=CARTESIAN_POINT ( 'NONE',  ( -120.4392612185200022, 1309.112692017090239, 300.3762800269190052 ) ) ;
#65776=CIRCLE ( 'NONE', #17443, 9.522913805090002626 ) ;
#65845=EDGE_CURVE ( 'NONE', #7591, #19696, #68781, .T. ) ;
#65897=CARTESIAN_POINT ( 'NONE',  ( -124.1574587856573828, 1375.179104070688027, 298.3450194382638756 ) ) ;
#66175=CARTESIAN_POINT ( 'NONE',  ( -118.9277976642162855, 1311.832804576488797, 294.9031044600987457 ) ) ;
#66454=CARTESIAN_POINT ( 'NONE',  ( -105.5311032031419956, 1320.102705746889569, 317.4872039844588016 ) ) ;
#66718=CARTESIAN_POINT ( 'NONE',  ( -96.14154407968888449, 1340.114449826970031, 304.2218459572590064 ) ) ;
#66841=ADVANCED_FACE ( 'NONE', ( #73708 ), #30575, .F. ) ;
#66866=EDGE_CURVE ( 'NONE', #89357, #10275, #88257, .T. ) ;
#66884=VECTOR ( 'NONE', #49798, 1000.000000000000114 ) ;
#66995=CARTESIAN_POINT ( 'NONE',  ( -107.0031525618482107, 1366.350733876290633, 315.0056284496591275 ) ) ;
#67164=CARTESIAN_POINT ( 'NONE',  ( -104.0419184278400024, 1314.643966242390206, 309.3341892202889767 ) ) ;
#67269=CARTESIAN_POINT ( 'NONE',  ( -101.7585531838400357, 1320.102705746892298, 310.5815974945691096 ) ) ;
#67404=CARTESIAN_POINT ( 'NONE',  ( -123.7789942036000070, 1376.302340817389904, 298.5517755817790544 ) ) ;
#67425=DIRECTION ( 'NONE',  ( -4.648609652910299899E-17, -1.000000000000000000, 2.252106476759999926E-16 ) ) ;
#67550=CARTESIAN_POINT ( 'NONE',  ( -130.6584559203110416, 1340.114449826970940, 321.4803018775702412 ) ) ;
#67646=CIRCLE ( 'NONE', #92715, 3.000000000000002665 ) ;
#67886=EDGE_LOOP ( 'NONE', ( #105993, #34339, #70986, #109290, #24911 ) ) ;
#67999=ADVANCED_BREP_SHAPE_REPRESENTATION ( '', ( #46097, #21632 ), #71657 ) ;
#68107=CARTESIAN_POINT ( 'NONE',  ( -113.4000000000000057, 1311.832804576489934, 313.5405874544189828 ) ) ;
#68239=CARTESIAN_POINT ( 'NONE',  ( -113.4000000000000057, 1305.913060387289988, 304.2218459572590064 ) ) ;
#68241=AXIS2_PLACEMENT_3D ( 'NONE', #16321, #76814, #52726 ) ;
#68652=CARTESIAN_POINT ( 'NONE',  ( -120.4392612185250044, 1309.112692017090694, 300.3762800269186641 ) ) ;
#68781=CIRCLE ( 'NONE', #59817, 4.000000000000003553 ) ;
#68929=CARTESIAN_POINT ( 'NONE',  ( -106.6287828259400072, 1306.483669372790246, 297.4506287831988516 ) ) ;
#69069=DIRECTION ( 'NONE',  ( -1.836970198721029688E-16, -1.000000000000000000, 0.000000000000000000 ) ) ;
#69162=DIRECTION ( 'NONE',  ( -1.836970198721029688E-16, -1.000000000000000000, 0.000000000000000000 ) ) ;
#69459=DIRECTION ( 'NONE',  ( 4.057416247971030182E-16, 1.000000000000000000, -4.440892098500000003E-16 ) ) ;
#69478=CARTESIAN_POINT ( 'NONE',  ( -106.6287828259400357, 1306.483669372789791, 305.9508215967690603 ) ) ;
#69662=CONICAL_SURFACE ( 'NONE', #24835, 0.9999999999999956701, 0.7853981633970000820 ) ;
#69766=LINE ( 'NONE', #1429, #101636 ) ;
#70212=FILL_AREA_STYLE ('',( #89168 ) ) ;
#70390=DIRECTION ( 'NONE',  ( -0.6205445805634668410, -0.7071067811868649855, -0.3390050494208925458 ) ) ;
#70534=EDGE_LOOP ( 'NONE', ( #36160, #251, #98227, #4283 ) ) ;
#70536=AXIS2_PLACEMENT_3D ( 'NONE', #829, #26555, #286 ) ;
#70592=FACE_OUTER_BOUND ( 'NONE', #83664, .T. ) ;
#70639=EDGE_CURVE ( 'NONE', #32152, #81044, #110760, .T. ) ;
#70986=ORIENTED_EDGE ( 'NONE', *, *, #47971, .F. ) ;
#71288=CARTESIAN_POINT ( 'NONE',  ( -123.2094608543013834, 1377.418846546388522, 298.8629130685377504 ) ) ;
#71653=PLANE ( 'NONE',  #1026 ) ;
#71657=( GEOMETRIC_REPRESENTATION_CONTEXT ( 3 ) GLOBAL_UNCERTAINTY_ASSIGNED_CONTEXT ( ( #35647 ) ) GLOBAL_UNIT_ASSIGNED_CONTEXT ( ( #229, #36560, #37111 ) ) REPRESENTATION_CONTEXT ( 'NONE', 'WORKASPACE' ) );
#71844=CARTESIAN_POINT ( 'NONE',  ( -119.5163997959657820, 1378.528619065190696, 293.9108410952588315 ) ) ;
#71870=( NAMED_UNIT ( * ) PLANE_ANGLE_UNIT ( ) SI_UNIT ( $, .RADIAN. ) );
#72112=CARTESIAN_POINT ( 'NONE',  ( -102.6425412143391469, 1375.179104070689618, 310.0986724762475433 ) ) ;
#72365=CARTESIAN_POINT ( 'NONE',  ( -113.4000000000000057, 1376.302340817389904, 292.3950450905590515 ) ) ;
#72497=ORIENTED_EDGE ( 'NONE', *, *, #55500, .F. ) ;
#72628=ORIENTED_EDGE ( 'NONE', *, *, #47971, .T. ) ;
#73124=DIRECTION ( 'NONE',  ( -1.836970198721029688E-16, -1.000000000000000000, 0.000000000000000000 ) ) ;
#73461=CARTESIAN_POINT ( 'NONE',  ( -107.1941519259529798, 1348.229899472569514, 298.0159978832118099 ) ) ;
#73484=PRODUCT_CONTEXT ( 'NONE', #83513, 'mechanical' ) ;
#73706=CARTESIAN_POINT ( 'NONE',  ( -121.7571430937320827, 1378.913060387289988, 299.6563178771723415 ) ) ;
#73708=FACE_OUTER_BOUND ( 'NONE', #80918, .T. ) ;
#73747=CARTESIAN_POINT ( 'NONE',  ( -123.7789942035663557, 1376.302340817389450, 298.5517755817776333 ) ) ;
#73768=VERTEX_POINT ( 'NONE', #104687 ) ;
#73821=DIRECTION ( 'NONE',  ( 0.6038592750913979179, 0.7071067811868638753, -0.3679048462383226470 ) ) ;
#73897=CARTESIAN_POINT ( 'NONE',  ( -112.5224174381096276, 1308.913060387289988, 304.7012714958631818 ) ) ;
#74005=CARTESIAN_POINT ( 'NONE',  ( -119.7254833230812636, 1314.643966242390889, 293.5583688343593280 ) ) ;
#74067=CARTESIAN_POINT ( 'NONE',  ( -107.4576978852700080, 1306.483669372790018, 307.4681403979390097 ) ) ;
#74167=AXIS2_PLACEMENT_3D ( 'NONE', #55779, #12085, #97745 ) ;
#74560=CARTESIAN_POINT ( 'NONE',  ( -96.21470915085022568, 1331.448250124730293, 308.6099712340398469 ) ) ;
#74843=CARTESIAN_POINT ( 'NONE',  ( -101.7585531180924079, 1320.102705746889797, 310.5815973742185747 ) ) ;
#74966=ADVANCED_FACE ( 'NONE', ( #20974 ), #42838, .T. ) ;
#75065=CIRCLE ( 'NONE', #57171, 4.000000000000003553 ) ;
#75114=CARTESIAN_POINT ( 'NONE',  ( -113.4000000000000057, 1320.102705746890251, 290.9564879300589837 ) ) ;
#75180=DIRECTION ( 'NONE',  ( -1.836970198721029688E-16, -1.000000000000000000, 0.000000000000000000 ) ) ;
#75397=CARTESIAN_POINT ( 'NONE',  ( -107.9538559484733327, 1348.229899472569059, 307.1970880126511929 ) ) ;
#75659=CARTESIAN_POINT ( 'NONE',  ( -96.21470915085019726, 1331.448250124730066, 304.2218459572590064 ) ) ;
#75738=CARTESIAN_POINT ( 'NONE',  ( -113.4000000000000057, 1306.483669372790018, 304.2218459572590064 ) ) ;
#75784=CARTESIAN_POINT ( 'NONE',  ( -124.7066708633999923, 1371.894749952190068, 298.0449835127589608 ) ) ;
#75821=EDGE_LOOP ( 'NONE', ( #91303, #51534, #88509, #50073 ) ) ;
#75927=CARTESIAN_POINT ( 'NONE',  ( -103.2058326176597376, 1331.448250124730066, 321.4071368064087437 ) ) ;
#76475=CARTESIAN_POINT ( 'NONE',  ( -104.3512419375300055, 1378.528619065190014, 309.1652050167789980 ) ) ;
#76477=CARTESIAN_POINT ( 'NONE',  ( -103.9363405334473356, 1366.350733876288359, 309.3918666868620448 ) ) ;
#76500=COLOUR_RGB ( '', 0.09019608, 0.27058824, 0.51372549) ;
#76644=CARTESIAN_POINT ( 'NONE',  ( -102.6425412143000102, 1375.179104070690073, 310.0986724762790345 ) ) ;
#76814=DIRECTION ( 'NONE',  ( 9.404037925578970303E-16, -1.000000000000000000, 2.220446049250000002E-16 ) ) ;
#76834=ADVANCED_FACE ( 'NONE', ( #70592 ), #89435, .T. ) ;
#76894=CARTESIAN_POINT ( 'NONE',  ( -122.7580815721600089, 1314.643966242390206, 299.1095026942290360 ) ) ;
#77042=CARTESIAN_POINT ( 'NONE',  ( -124.0634771228999966, 1314.643966242390206, 304.2218459572590064 ) ) ;
#77117=DIRECTION ( 'NONE',  ( -1.836970198721029688E-16, -1.000000000000000000, -1.314768175368352060E-31 ) ) ;
#77175=DIRECTION ( 'NONE',  ( -1.000000000000000000, 0.000000000000000000, 0.000000000000000000 ) ) ;
#77300=VERTEX_POINT ( 'NONE', #40274 ) ;
#77810=DIRECTION ( 'NONE',  ( -1.836970198721029688E-16, -1.000000000000000000, 0.000000000000000000 ) ) ;
#78405=CARTESIAN_POINT ( 'NONE',  ( -105.3788045886400084, 1309.112692017090239, 304.2218459572590064 ) ) ;
#78804=FACE_OUTER_BOUND ( 'NONE', #37924, .T. ) ;
#79254=CARTESIAN_POINT ( 'NONE',  ( -109.3833719510217293, 1306.483669372788654, 310.9930631313186495 ) ) ;
#79663=CARTESIAN_POINT ( 'NONE',  ( -102.2221789262000016, 1377.418846546390114, 304.2218459572590064 ) ) ;
#80197=CARTESIAN_POINT ( 'NONE',  ( -101.1419410403000256, 1375.179104070690528, 307.3518423499588152 ) ) ;
#80223=( LENGTH_UNIT ( ) NAMED_UNIT ( * ) SI_UNIT ( .MILLI., .METRE. ) );
#80662=CIRCLE ( 'NONE', #62803, 5.868098490439995985 ) ;
#80749=CARTESIAN_POINT ( 'NONE',  ( -120.6713756150341652, 1375.179104070688936, 291.9637869975590547 ) ) ;
#80776=( NAMED_UNIT ( * ) SI_UNIT ( $, .STERADIAN. ) SOLID_ANGLE_UNIT ( ) );
#80783=EDGE_LOOP ( 'NONE', ( #17505, #54847, #38195, #14643 ) ) ;
#80918=EDGE_LOOP ( 'NONE', ( #56466, #62100, #12466, #5523, #42318 ) ) ;
#81023=CARTESIAN_POINT ( 'NONE',  ( -102.0933291365972053, 1371.894749952189159, 310.3987084017696816 ) ) ;
#81044=VERTEX_POINT ( 'NONE', #14451 ) ;
#81096=EDGE_LOOP ( 'NONE', ( #72497, #98301, #29747, #58882 ) ) ;
#81277=CARTESIAN_POINT ( 'NONE',  ( -113.4000000000000057, 1371.894749952190068, 291.3379631701589574 ) ) ;
#81447=ORIENTED_EDGE ( 'NONE', *, *, #53107, .F. ) ;
#81827=CARTESIAN_POINT ( 'NONE',  ( -107.9538559792320740, 1348.229899472569059, 307.1970880689542582 ) ) ;
#82116=CARTESIAN_POINT ( 'NONE',  ( -124.5778210737999956, 1377.418846546390114, 304.2218459572590064 ) ) ;
#82319=EDGE_CURVE ( 'NONE', #17543, #38227, #42631, .T. ) ;
#82401=CARTESIAN_POINT ( 'NONE',  ( -121.2688967968579448, 1320.102705746890251, 290.9564879300592679 ) ) ;
#82679=CARTESIAN_POINT ( 'NONE',  ( -113.4000000000000057, 1378.528619065190014, 314.5328508192589538 ) ) ;
#82937=CARTESIAN_POINT ( 'NONE',  ( -102.7365228770999295, 1314.643966242389752, 293.5583688343589301 ) ) ;
#83227=CARTESIAN_POINT ( 'NONE',  ( -109.2808341013028297, 1358.631207110788409, 311.1659210709986496 ) ) ;
#83350=CARTESIAN_POINT ( 'NONE',  ( -113.4000000000000057, 1306.913060387289988, 304.2218459572590064 ) ) ;
#83479=CARTESIAN_POINT ( 'NONE',  ( -113.4000000000000057, 1314.643966242390206, 293.5583688343590438 ) ) ;
#83513=APPLICATION_CONTEXT ( 'automotive_design' ) ;
#83664=EDGE_LOOP ( 'NONE', ( #81447, #47987, #22482, #3988 ) ) ;
#83776=CARTESIAN_POINT ( 'NONE',  ( -128.4815115702291735, 1331.448250124730521, 295.9827786358369508 ) ) ;
#83904=DIRECTION ( 'NONE',  ( -1.836970198721029688E-16, -1.000000000000000000, 0.000000000000000000 ) ) ;
#84038=CARTESIAN_POINT ( 'NONE',  ( -102.6162175075999556, 1366.350733876290860, 306.9753977562709224 ) ) ;
#84168=CARTESIAN_POINT ( 'NONE',  ( -123.8569892973000037, 1368.558218059089995, 298.5091666678990237 ) ) ;
#84323=CARTESIAN_POINT ( 'NONE',  ( -119.6058480740470600, 1348.229899472569514, 310.4276940313061459 ) ) ;
#84567=FACE_OUTER_BOUND ( 'NONE', #67886, .T. ) ;
#84857=CARTESIAN_POINT ( 'NONE',  ( -130.5852908491498852, 1331.448250124730066, 299.8337207750958555 ) ) ;
#85134=CARTESIAN_POINT ( 'NONE',  ( -119.3423021147299607, 1306.483669372790018, 300.9755515165832662 ) ) ;
#85408=CARTESIAN_POINT ( 'NONE',  ( -107.3060007717225375, 1358.631207110789546, 307.5510129087674045 ) ) ;
#85578=CARTESIAN_POINT ( 'NONE',  ( -103.9363405334299983, 1366.350733876289951, 309.3918666868790410 ) ) ;
#85882=DIRECTION ( 'NONE',  ( -1.000000000000000000, 0.000000000000000000, 0.000000000000000000 ) ) ;
#86053=DIRECTION ( 'NONE',  ( 0.8775825618903687619, 0.000000000000000000, 0.4794255386042102218 ) ) ;
#86674=DIRECTION ( 'NONE',  ( -1.836970198721029688E-16, -1.000000000000000000, 0.000000000000000000 ) ) ;
#86919=AXIS2_PLACEMENT_3D ( 'NONE', #34541, #77117, #86053 ) ;
#87056=EDGE_LOOP ( 'NONE', ( #39568, #15582, #40841, #103523 ) ) ;
#87490=CARTESIAN_POINT ( 'NONE',  ( -113.4000000000000057, 1308.913060387289988, 304.2218459572590064 ) ) ;
#87504=CARTESIAN_POINT ( 'NONE',  ( -102.9430107618170069, 1368.558218059089086, 309.9345253547082280 ) ) ;
#87531=PRODUCT_DEFINITION_SHAPE ( 'NONE', 'NONE',  #11756 ) ;
#87654=PRESENTATION_STYLE_ASSIGNMENT (( #97147 ) ) ;
#87789=CARTESIAN_POINT ( 'NONE',  ( -113.4000000000000057, 1377.913060387289988, 304.2218459572590064 ) ) ;
#87845=DIRECTION ( 'NONE',  ( -0.8539859765994315399, 0.000000000000000000, 0.5202960232132425311 ) ) ;
#88064=CARTESIAN_POINT ( 'NONE',  ( -103.0889951380000014, 1378.528619065189559, 306.8546778052111108 ) ) ;
#88257=CIRCLE ( 'NONE', #107904, 4.000000000000003553 ) ;
#88470=DIRECTION ( 'NONE',  ( -4.222254822704919979E-17, -1.000000000000000000, 7.728785610902649958E-17 ) ) ;
#88509=ORIENTED_EDGE ( 'NONE', *, *, #20435, .T. ) ;
#88610=CARTESIAN_POINT ( 'NONE',  ( -120.4155570069220431, 1376.302340817389222, 292.3950450905591083 ) ) ;
#88718=CARTESIAN_POINT ( 'NONE',  ( -113.4000000000000057, 1377.913060387289988, 304.2218459572590064 ) ) ;
#88877=CARTESIAN_POINT ( 'NONE',  ( -113.4000000000000057, 1375.179104070690073, 316.4799049169590148 ) ) ;
#89143=CARTESIAN_POINT ( 'NONE',  ( -101.1419410402999972, 1375.179104070690073, 304.2218459572590064 ) ) ;
#89168=FILL_AREA_STYLE_COLOUR ( '', #91520 ) ;
#89177=ORIENTED_EDGE ( 'NONE', *, *, #10464, .T. ) ;
#89285=CONICAL_SURFACE ( 'NONE', #41003, 0.9999999999999930056, 0.7853981633970000820 ) ;
#89357=VERTEX_POINT ( 'NONE', #56852 ) ;
#89425=CARTESIAN_POINT ( 'NONE',  ( -105.7573910491803844, 1371.894749952187794, 317.1057287443589985 ) ) ;
#89435=TOROIDAL_SURFACE ( 'NONE', #96631, 5.868098490439999537, 1.000000000000000000 ) ;
#89687=CARTESIAN_POINT ( 'NONE',  ( -121.0426089508195560, 1371.894749952188249, 291.3379631701592416 ) ) ;
#89737=AXIS2_PLACEMENT_3D ( 'NONE', #102087, #67425, #101524 ) ;
#89773=AXIS2_PLACEMENT_3D ( 'NONE', #83350, #83904, #109129 ) ;
#89800=DIRECTION ( 'NONE',  ( 0.8775825618903746461, -8.693568535565067726E-32, 0.4794255386041995082 ) ) ;
#89840=SURFACE_SIDE_STYLE ('',( #63041 ) ) ;
#90226=CARTESIAN_POINT ( 'NONE',  ( -101.4843241976999906, 1368.558218059089995, 304.2218459572590064 ) ) ;
#90237=AXIS2_PLACEMENT_3D ( 'NONE', #65303, #99414, #14862 ) ;
#90574=CARTESIAN_POINT ( 'NONE',  ( -118.5497409066653773, 1306.913060387289988, 301.4085296778973202 ) ) ;
#90747=DIRECTION ( 'NONE',  ( -1.000000000000000000, 0.000000000000000000, 0.000000000000000000 ) ) ;
#90786=CARTESIAN_POINT ( 'NONE',  ( -128.5457199608244139, 1340.114449826971168, 295.9477014321976753 ) ) ;
#90859=CARTESIAN_POINT ( 'NONE',  ( -116.0327476856711257, 1378.813060387289852, 302.7835693414463663 ) ) ;
#91066=CARTESIAN_POINT ( 'NONE',  ( -122.4487580624584382, 1378.528619065188877, 299.2784868977452675 ) ) ;
#91303=ORIENTED_EDGE ( 'NONE', *, *, #102111, .F. ) ;
#91347=CARTESIAN_POINT ( 'NONE',  ( -119.4939992282775023, 1358.631207110791138, 300.8926790057503240 ) ) ;
#91421=DIRECTION ( 'NONE',  ( -1.000000000000000000, 0.000000000000000000, 0.000000000000000000 ) ) ;
#91434=DIRECTION ( 'NONE',  ( -1.000000000000000000, 0.000000000000000000, 0.000000000000000000 ) ) ;
#91480=CARTESIAN_POINT ( 'NONE',  ( -123.2094608543100094, 1377.418846546390114, 298.8629130685190489 ) ) ;
#91520=COLOUR_RGB ( '', 0.09019608, 0.27058824, 0.51372549) ;
#91525=ADVANCED_FACE ( 'NONE', ( #37207 ), #46724, .T. ) ;
#91624=CARTESIAN_POINT ( 'NONE',  ( -124.0634771228999682, 1314.643966242389070, 301.4990132218018175 ) ) ;
#91888=CARTESIAN_POINT ( 'NONE',  ( -123.8569892972415545, 1368.558218059090223, 298.5091666679153946 ) ) ;
#92177=CARTESIAN_POINT ( 'NONE',  ( -130.5852908491499988, 1331.448250124730066, 304.2218459572590064 ) ) ;
#92218=( BOUNDED_SURFACE ( )  B_SPLINE_SURFACE ( 5, 2, ( 
 ( #97008, #88064, #63969, #29782, #20271, #71844, #105962 ),
 ( #63429, #12969, #79663, #20819, #2967, #54472, #71288 ),
 ( #105401, #55016, #98084, #11349, #72365, #88610, #46064 ),
 ( #21355, #80197, #89143, #12429, #44964, #80749, #106496 ),
 ( #55562, #107042, #64518, #4058, #81277, #89687, #53359 ),
 ( #87504, #65612, #90226, #15161, #5130, #24111, #91888 ),
 ( #33078, #84038, #13511, #47699, #99724, #48815, #30877 ),
 ( #23017, #99170, #65057, #22452, #14069, #57221, #91347 ),
 ( #81827, #31430, #58303, #73461, #7336, #49903, #39286 ),
 ( #14628, #107592, #66718, #41500, #5697, #56653, #90786 ),
 ( #32545, #74560, #75659, #6772, #92425, #108137, #109800 ),
 ( #67269, #100824, #40936, #48258, #75114, #82401, #40383 ),
 ( #15700, #39842, #21901, #82937, #83479, #74005, #6228 ),
 ( #109261, #49352, #108693, #56098, #31985, #66175, #100295 ),
 ( #23576, #57769, #78405, #60518, #25213, #35856, #51003 ),
 ( #34739, #69478, #102481, #68929, #1717, #51549, #85134 ) ),
 .UNSPECIFIED., .F., .F., .F. ) 
 B_SPLINE_SURFACE_WITH_KNOTS ( ( 6, 3, 3, 1, 3, 6 ),
 ( 3, 2, 2, 3 ),
 ( 0.4214913904879999951, 6.500000000000000000, 18.08975840989999995, 46.86861349480000172, 60.45619974110000072, 75.86994138869999915 ),
 ( 5.770213214419189995, 6.283185307179590673, 7.853981633974480125, 8.911805878012440729 ),
 .UNSPECIFIED. ) 
 GEOMETRIC_REPRESENTATION_ITEM ( )  RATIONAL_B_SPLINE_SURFACE ( (
 ( 0.8711730249283579086, 0.9043503954986760185, 1.000000000000000000, 0.7071067811865480168, 1.000000000000000000, 0.8027563838226109416, 0.8711730262223410515),
 ( 0.8711730249283579086, 0.9043503954986760185, 1.000000000000000000, 0.7071067811865480168, 1.000000000000000000, 0.8027563838226109416, 0.8711730262223410515),
 ( 0.8711730249283579086, 0.9043503954986760185, 1.000000000000000000, 0.7071067811865480168, 1.000000000000000000, 0.8027563838226109416, 0.8711730262223410515),
 ( 0.8711730249283579086, 0.9043503954986760185, 1.000000000000000000, 0.7071067811865480168, 1.000000000000000000, 0.8027563838226109416, 0.8711730262223410515),
 ( 0.8711730249283579086, 0.9043503954986760185, 1.000000000000000000, 0.7071067811865480168, 1.000000000000000000, 0.8027563838226109416, 0.8711730262223410515),
 ( 0.8711730249283579086, 0.9043503954986760185, 1.000000000000000000, 0.7071067811865480168, 1.000000000000000000, 0.8027563838226109416, 0.8711730262223410515),
 ( 0.8711730249283579086, 0.9043503954986760185, 1.000000000000000000, 0.7071067811865480168, 1.000000000000000000, 0.8027563838226109416, 0.8711730262223410515),
 ( 0.8711730249283579086, 0.9043503954986760185, 1.000000000000000000, 0.7071067811865480168, 1.000000000000000000, 0.8027563838226109416, 0.8711730262223410515),
 ( 0.8711730249283579086, 0.9043503954986760185, 1.000000000000000000, 0.7071067811865480168, 1.000000000000000000, 0.8027563838226109416, 0.8711730262223410515),
 ( 0.8711730249283579086, 0.9043503954986760185, 1.000000000000000000, 0.7071067811865480168, 1.000000000000000000, 0.8027563838226109416, 0.8711730262223410515),
 ( 0.8711730249283579086, 0.9043503954986760185, 1.000000000000000000, 0.7071067811865480168, 1.000000000000000000, 0.8027563838226109416, 0.8711730262223410515),
 ( 0.8711730249283579086, 0.9043503954986760185, 1.000000000000000000, 0.7071067811865480168, 1.000000000000000000, 0.8027563838226109416, 0.8711730262223410515),
 ( 0.8711730249283579086, 0.9043503954986760185, 1.000000000000000000, 0.7071067811865480168, 1.000000000000000000, 0.8027563838226109416, 0.8711730262223410515),
 ( 0.8711730249283579086, 0.9043503954986760185, 1.000000000000000000, 0.7071067811865480168, 1.000000000000000000, 0.8027563838226109416, 0.8711730262223410515),
 ( 0.8711730249283579086, 0.9043503954986760185, 1.000000000000000000, 0.7071067811865480168, 1.000000000000000000, 0.8027563838226109416, 0.8711730262223410515),
 ( 0.8711730249283579086, 0.9043503954986760185, 1.000000000000000000, 0.7071067811865480168, 1.000000000000000000, 0.8027563838226109416, 0.8711730262223410515) ) ) 
 REPRESENTATION_ITEM ( '' )  SURFACE ( )  );
#92370=ADVANCED_FACE ( 'NONE', ( #84567 ), #27122, .F. ) ;
#92425=CARTESIAN_POINT ( 'NONE',  ( -113.4000000000000057, 1331.448250124730066, 287.0365551081090416 ) ) ;
#92465=AXIS2_PLACEMENT_3D ( 'NONE', #27847, #18866, #8815 ) ;
#92564=CARTESIAN_POINT ( 'NONE',  ( -121.5779650366699940, 1311.832804576489934, 299.7542032958689902 ) ) ;
#92715=AXIS2_PLACEMENT_3D ( 'NONE', #102653, #7518, #85882 ) ;
#92719=CARTESIAN_POINT ( 'NONE',  ( -122.7580815721744614, 1314.643966242390661, 299.1095026942199411 ) ) ;
#92795=UNCERTAINTY_MEASURE_WITH_UNIT (LENGTH_MEASURE( 1.000000000000000082E-05 ), #4196, 'distance_accuracy_value', 'NONE');
#93272=CARTESIAN_POINT ( 'NONE',  ( -120.3440751137400895, 1358.631207110788864, 302.4487324766139409 ) ) ;
#93325=ADVANCED_FACE ( 'NONE', ( #53929 ), #92218, .T. ) ;
#93623=EDGE_CURVE ( 'NONE', #41956, #44860, #46881, .T. ) ;
#93804=CARTESIAN_POINT ( 'NONE',  ( -124.1837824924000557, 1366.350733876289723, 315.0056284496589001 ) ) ;
#94148=FACE_OUTER_BOUND ( 'NONE', #56355, .T. ) ;
#94158=EDGE_CURVE ( 'NONE', #73768, #26502, #80662, .T. ) ;
#94224=CARTESIAN_POINT ( 'NONE',  ( -113.4000000000000057, 1378.528619065190014, 304.2218459572590064 ) ) ;
#95080=ORIENTED_EDGE ( 'NONE', *, *, #33145, .F. ) ;
#95430=FACE_OUTER_BOUND ( 'NONE', #70534, .T. ) ;
#95557=CYLINDRICAL_SURFACE ( 'NONE', #86919, 3.000000000000017764 ) ;
#96036=CARTESIAN_POINT ( 'NONE',  ( -108.6418955636174672, 1309.112692017088193, 312.2430413686188331 ) ) ;
#96631=AXIS2_PLACEMENT_3D ( 'NONE', #62188, #88470, #19593 ) ;
#96882=DIRECTION ( 'NONE',  ( 0.8775825618903754233, 0.000000000000000000, 0.4794255386041978984 ) ) ;
#97008=CARTESIAN_POINT ( 'NONE',  ( -104.3512419886430109, 1378.528619065190469, 309.1652051103151848 ) ) ;
#97033=SURFACE_STYLE_USAGE ( .BOTH. , #53953 ) ;
#97112=DIRECTION ( 'NONE',  ( -4.222254822704964968E-17, -1.000000000000000000, 7.728785610902679540E-17 ) ) ;
#97147=SURFACE_STYLE_USAGE ( .BOTH. , #89840 ) ;
#97598=ORIENTED_EDGE ( 'NONE', *, *, #66866, .F. ) ;
#97745=DIRECTION ( 'NONE',  ( -0.8775825618903754233, 0.000000000000000000, -0.4794255386041978984 ) ) ;
#97813=CARTESIAN_POINT ( 'NONE',  ( -113.4000000000000057, 1371.894749952190068, 317.1057287443589985 ) ) ;
#98059=ADVANCED_FACE ( 'NONE', ( #35686, #78804 ), #9933, .T. ) ;
#98084=CARTESIAN_POINT ( 'NONE',  ( -101.5731991332999939, 1376.302340817389904, 304.2218459572590064 ) ) ;
#98177=DIRECTION ( 'NONE',  ( -1.000000000000000000, 0.000000000000000000, 0.000000000000000000 ) ) ;
#98227=ORIENTED_EDGE ( 'NONE', *, *, #94158, .F. ) ;
#98301=ORIENTED_EDGE ( 'NONE', *, *, #65595, .T. ) ;
#98798=DIRECTION ( 'NONE',  ( -4.222254822704964968E-17, -1.000000000000000000, 7.728785610902679540E-17 ) ) ;
#98915=CARTESIAN_POINT ( 'NONE',  ( -123.7110048619999958, 1378.528619065190014, 304.2218459572590064 ) ) ;
#99170=CARTESIAN_POINT ( 'NONE',  ( -106.4559248862600214, 1358.631207110789319, 305.9949594761371827 ) ) ;
#99414=DIRECTION ( 'NONE',  ( -1.836970198721029688E-16, -1.000000000000000000, -1.314768175368352060E-31 ) ) ;
#99457=CARTESIAN_POINT ( 'NONE',  ( -106.3844429930778972, 1376.302340817388313, 316.0486468239590181 ) ) ;
#99724=CARTESIAN_POINT ( 'NONE',  ( -113.4000000000000057, 1366.350733876289951, 293.4380634648589989 ) ) ;
#100014=CARTESIAN_POINT ( 'NONE',  ( -125.6580589596999999, 1375.179104070690073, 304.2218459572590064 ) ) ;
#100295=CARTESIAN_POINT ( 'NONE',  ( -121.5779650366748399, 1311.832804576490162, 299.7542032958752998 ) ) ;
#100567=CARTESIAN_POINT ( 'NONE',  ( -122.7187414971599964, 1311.832804576489934, 304.2218459572590064 ) ) ;
#100824=CARTESIAN_POINT ( 'NONE',  ( -100.1346419727999972, 1320.102705746889797, 307.6090480346439904 ) ) ;
#100960=CARTESIAN_POINT ( 'NONE',  ( -119.3423021147300034, 1306.483669372790018, 300.9755515165790030 ) ) ;
#101105=CARTESIAN_POINT ( 'NONE',  ( -113.4000000000000057, 1348.229899472569969, 310.4276940313059754 ) ) ;
#101261=CARTESIAN_POINT ( 'NONE',  ( -103.0210057964000043, 1376.302340817389904, 309.8919163327390152 ) ) ;
#101524=DIRECTION ( 'NONE',  ( -1.000000000000000000, 0.000000000000000000, 0.000000000000000000 ) ) ;
#101636=VECTOR ( 'NONE', #8706, 1000.000000000000000 ) ;
#101652=CARTESIAN_POINT ( 'NONE',  ( -104.0419184278224094, 1314.643966242388842, 309.3341892202922168 ) ) ;
#102066=CARTESIAN_POINT ( 'NONE',  ( -126.7681019193000225, 1325.797319984390015, 296.9188185942790028 ) ) ;
#102087=CARTESIAN_POINT ( 'NONE',  ( -113.4000000000000057, 1377.913060387289988, 304.2218459572590064 ) ) ;
#102111=EDGE_CURVE ( 'NONE', #20038, #17543, #21151, .T. ) ;
#102222=CARTESIAN_POINT ( 'NONE',  ( -105.2220349633250862, 1311.832804576488797, 308.6894886186424856 ) ) ;
#102438=DIRECTION ( 'NONE',  ( -1.000000000000000000, 0.000000000000000000, 0.000000000000000000 ) ) ;
#102481=CARTESIAN_POINT ( 'NONE',  ( -106.6287828259400072, 1306.483669372790018, 304.2218459572590064 ) ) ;
#102653=CARTESIAN_POINT ( 'NONE',  ( -113.4000000000000057, 1306.913060387289988, 304.2218459572590064 ) ) ;
#102685=TOROIDAL_SURFACE ( 'NONE', #70536, 5.868098490439999537, 1.000000000000000000 ) ;
#103148=DIRECTION ( 'NONE',  ( 0.8775825618903754233, 0.000000000000000000, 0.4794255386041978984 ) ) ;
#103281=ORIENTED_EDGE ( 'NONE', *, *, #12558, .F. ) ;
#103523=ORIENTED_EDGE ( 'NONE', *, *, #10464, .F. ) ;
#103639=ADVANCED_FACE ( 'NONE', ( #62101 ), #69662, .F. ) ;
#103830=CIRCLE ( 'NONE', #101, 9.522913805090002626 ) ;
#103884=CARTESIAN_POINT ( 'NONE',  ( -121.4211954113599745, 1309.112692017089785, 312.2430413686192310 ) ) ;
#104036=CIRCLE ( 'NONE', #89737, 3.000000000000002665 ) ;
#104438=CARTESIAN_POINT ( 'NONE',  ( -119.3423021147281418, 1306.483669372790018, 300.9755515165800830 ) ) ;
#104687=CARTESIAN_POINT ( 'NONE',  ( -108.2502590933346198, 1305.913060387290216, 307.0351622366206357 ) ) ;
#104692=ORIENTED_EDGE ( 'NONE', *, *, #104815, .F. ) ;
#104815=EDGE_CURVE ( 'NONE', #41956, #10275, #36206, .T. ) ;
#105278=EDGE_CURVE ( 'NONE', #10275, #89357, #75065, .T. ) ;
#105401=CARTESIAN_POINT ( 'NONE',  ( -103.0210058550480738, 1376.302340817390359, 309.8919164400330146 ) ) ;
#105568=DIRECTION ( 'NONE',  ( 0.8775825618903746461, -8.693568535565067726E-32, 0.4794255386041995082 ) ) ;
#105962=CARTESIAN_POINT ( 'NONE',  ( -122.4487580624616498, 1378.528619065190014, 299.2784868977504402 ) ) ;
#105993=ORIENTED_EDGE ( 'NONE', *, *, #25444, .T. ) ;
#106098=FILL_AREA_STYLE ('',( #28846 ) ) ;
#106226=CARTESIAN_POINT ( 'NONE',  ( -104.3512419375385036, 1378.528619065190242, 309.1652050167673451 ) ) ;
#106482=B_SPLINE_CURVE_WITH_KNOTS ( 'NONE', 5,
 ( #7239, #49806, #17810, #67164, #52010, #16163, #41399, #17255, #34643, #40834, #32974, #85578, #6680, #15601, #76644, #101261, #50902, #33513 ),
 .UNSPECIFIED., .F., .F.,
 ( 6, 3, 3, 3, 3, 6 ),
 ( -75.86994138869999915, -60.45619974110000072, -46.86861349480000172, -18.08975840989999284, -6.500000000000000000, -0.4214913904880006612 ),
 .UNSPECIFIED. ) ;
#106496=CARTESIAN_POINT ( 'NONE',  ( -124.1574587856609071, 1375.179104070688936, 298.3450194382701852 ) ) ;
#106584=CARTESIAN_POINT ( 'NONE',  ( -113.4000000000000057, 1305.913060387289988, 304.2218459572590064 ) ) ;
#107042=CARTESIAN_POINT ( 'NONE',  ( -100.5161172128999993, 1371.894749952189613, 307.5116414118388093 ) ) ;
#107319=ORIENTED_EDGE ( 'NONE', *, *, #66866, .T. ) ;
#107324=CARTESIAN_POINT ( 'NONE',  ( -123.7110048619999958, 1378.528619065190696, 314.5328508192591244 ) ) ;
#107399=DIRECTION ( 'NONE',  ( -1.836970198721029688E-16, -1.000000000000000000, 0.000000000000000000 ) ) ;
#107527=CONICAL_SURFACE ( 'NONE', #68241, 0.9999999999999930056, 0.7853981633970000820 ) ;
#107592=CARTESIAN_POINT ( 'NONE',  ( -96.14154407968895555, 1340.114449826968894, 308.6286533442801101 ) ) ;
#107871=CARTESIAN_POINT ( 'NONE',  ( -125.2268008667000458, 1376.302340817389677, 316.0486468239593592 ) ) ;
#107904=AXIS2_PLACEMENT_3D ( 'NONE', #58550, #69162, #24899 ) ;
#107981=DIRECTION ( 'NONE',  ( -1.000000000000000000, 0.000000000000000000, 0.000000000000000000 ) ) ;
#108137=CARTESIAN_POINT ( 'NONE',  ( -123.5941673823403306, 1331.448250124728247, 287.0365551081088142 ) ) ;
#108277=EDGE_CURVE ( 'NONE', #77300, #20038, #103830, .T. ) ;
#108288=ORIENTED_EDGE ( 'NONE', *, *, #94158, .T. ) ;
#108423=EDGE_LOOP ( 'NONE', ( #97598, #35323 ) ) ;
#108539=CARTESIAN_POINT ( 'NONE',  ( -113.4000000000000057, 1377.913060387289988, 304.2218459572590064 ) ) ;
#108693=CARTESIAN_POINT ( 'NONE',  ( -104.0812585028400008, 1311.832804576489934, 304.2218459572590064 ) ) ;
#108708=MECHANICAL_DESIGN_GEOMETRIC_PRESENTATION_REPRESENTATION('',(#28228),#12158);
#108987=CARTESIAN_POINT ( 'NONE',  ( -113.4000000000000057, 1368.558218059089995, 316.1375217595589788 ) ) ;
#109079=ORIENTED_EDGE ( 'NONE', *, *, #29511, .F. ) ;
#109129=DIRECTION ( 'NONE',  ( -1.000000000000000000, 0.000000000000000000, 0.000000000000000000 ) ) ;
#109208=CARTESIAN_POINT ( 'NONE',  ( -118.5497409066653773, 1305.913060387290216, 301.4085296778973202 ) ) ;
#109261=CARTESIAN_POINT ( 'NONE',  ( -105.2220350095120551, 1311.832804576489707, 308.6894887031868393 ) ) ;
#109290=ORIENTED_EDGE ( 'NONE', *, *, #30977, .F. ) ;
#109536=CARTESIAN_POINT ( 'NONE',  ( -102.9430107027584285, 1368.558218059088631, 309.9345252466023908 ) ) ;
#109800=CARTESIAN_POINT ( 'NONE',  ( -128.4815115702338915, 1331.448250124728247, 295.9827786358457615 ) ) ;
#110080=CARTESIAN_POINT ( 'NONE',  ( -113.4000000000000057, 1314.643966242390206, 314.8853230801589689 ) ) ;
#110085=CARTESIAN_POINT ( 'NONE',  ( 0.000000000000000000, 0.000000000000000000, 0.000000000000000000 ) ) ;
#110110=CARTESIAN_POINT ( 'NONE',  ( -116.0327476856711115, 1377.913060387289988, 302.7835693414463663 ) ) ;
#110630=CARTESIAN_POINT ( 'NONE',  ( -122.7187414971600674, 1311.832804576489934, 301.8423806000122909 ) ) ;
#110760=CIRCLE ( 'NONE', #10704, 3.000000000000002665 ) ;
ENDSEC;
END-ISO-10303-21;
